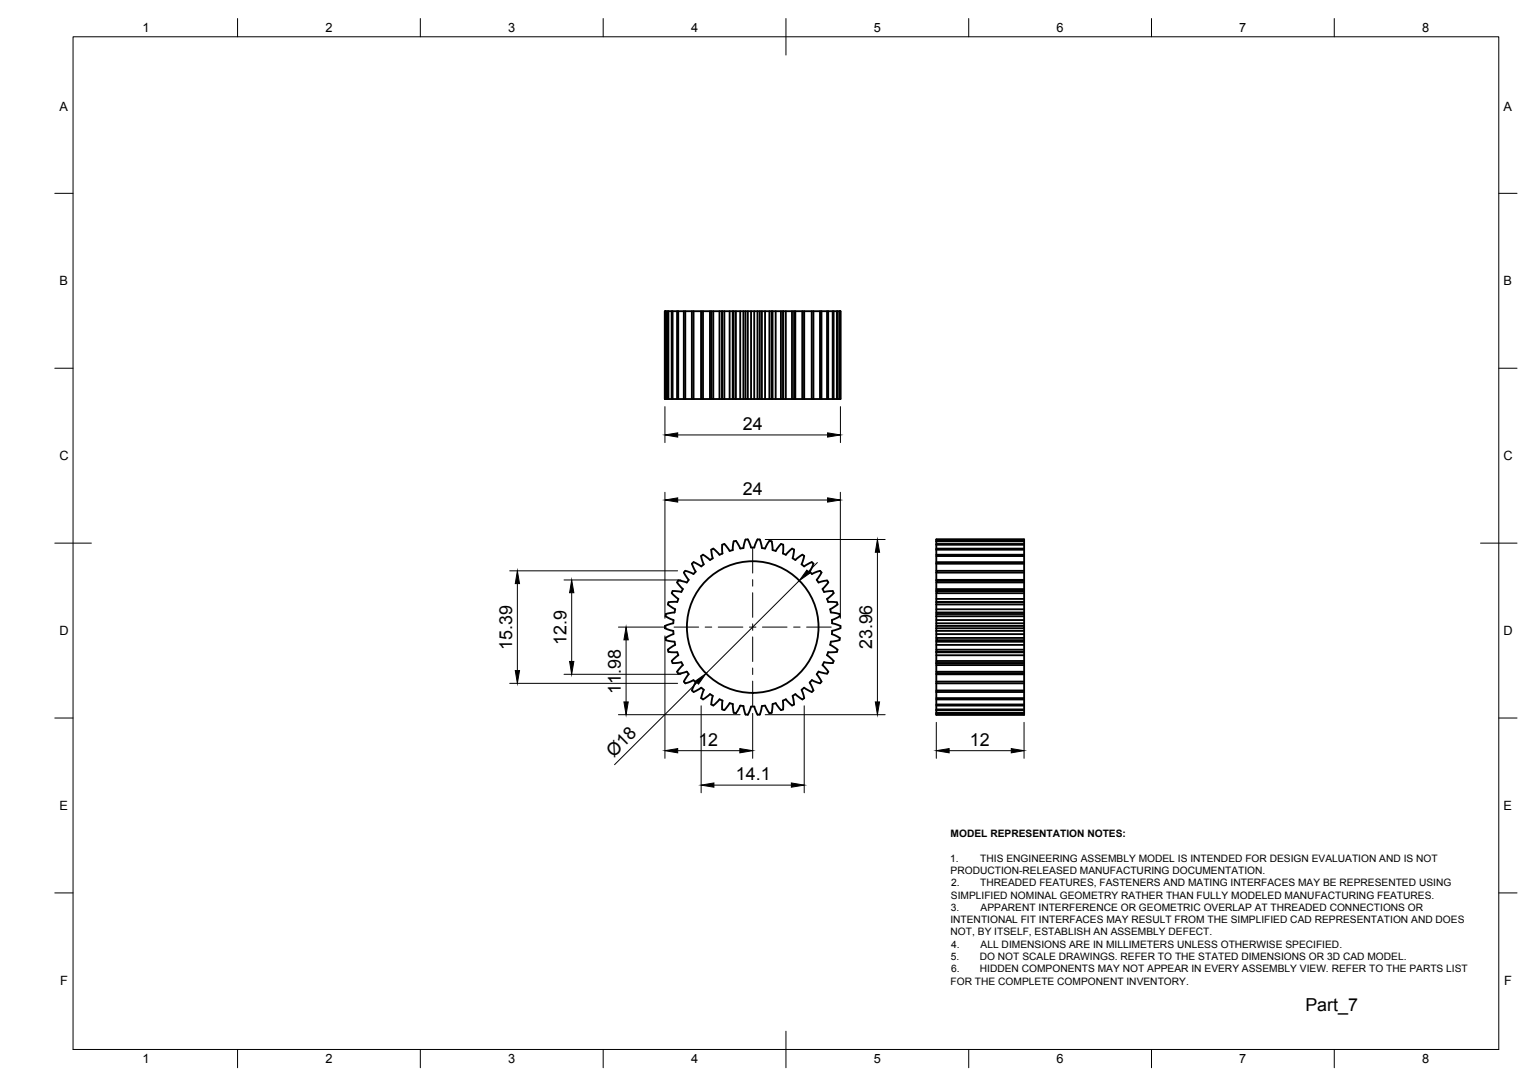
ISO-10303-21;
HEADER;
/* Generated by software containing ST-Developer
 * from STEP Tools, Inc. (www.steptools.com) 
 */

FILE_DESCRIPTION(
/* description */ ('STEP AP242 Edition 2'),
/* implementation_level */ '2;1');

FILE_NAME(
/* name */ 'Part_7.step',
/* time_stamp */ '2026-10-06T10:11:12-07:00',
/* author */ (''),
/* organization */ (''),
/* preprocessor_version */ 'ST-DEVELOPER v20.2',
/* originating_system */ 'Autodesk Translation Framework v15.15.0.0',
/* authorisation */ '');

FILE_SCHEMA (('AUTOMOTIVE_DESIGN { 1 0 10303 214 3 1 1 }'));
ENDSEC;

DATA;
#10=MECHANICAL_DESIGN_GEOMETRIC_PRESENTATION_REPRESENTATION('',(#1771),#54580);
#1743=SHAPE_REPRESENTATION_RELATIONSHIP('SRR','None',#54630,#1757);
#1757=ADVANCED_BREP_SHAPE_REPRESENTATION('',(#1801),#54566);
#1771=STYLED_ITEM('',(#54709),#1801);
#1801=MANIFOLD_SOLID_BREP('Body1',#17666);
#1815=LINE('',#24101,#2408);
#1816=LINE('',#24103,#2409);
#1817=LINE('',#24107,#2410);
#1818=LINE('',#24110,#2411);
#1819=LINE('',#24113,#2412);
#1820=LINE('',#24115,#2413);
#1821=LINE('',#24119,#2414);
#1822=LINE('',#24121,#2415);
#1823=LINE('',#24125,#2416);
#1824=LINE('',#24127,#2417);
#1825=LINE('',#24131,#2418);
#1826=LINE('',#24134,#2419);
#1827=LINE('',#24137,#2420);
#1828=LINE('',#24140,#2421);
#1829=LINE('',#24143,#2422);
#1830=LINE('',#24145,#2423);
#1831=LINE('',#24149,#2424);
#1832=LINE('',#24152,#2425);
#1833=LINE('',#24155,#2426);
#1834=LINE('',#24157,#2427);
#1835=LINE('',#24161,#2428);
#1836=LINE('',#24163,#2429);
#1837=LINE('',#24167,#2430);
#1838=LINE('',#24169,#2431);
#1839=LINE('',#24173,#2432);
#1840=LINE('',#24175,#2433);
#1841=LINE('',#24179,#2434);
#1842=LINE('',#24182,#2435);
#1843=LINE('',#24185,#2436);
#1844=LINE('',#24187,#2437);
#1845=LINE('',#24191,#2438);
#1846=LINE('',#24193,#2439);
#1847=LINE('',#24197,#2440);
#1848=LINE('',#24199,#2441);
#1849=LINE('',#24203,#2442);
#1850=LINE('',#24206,#2443);
#1851=LINE('',#24209,#2444);
#1852=LINE('',#24212,#2445);
#1853=LINE('',#24215,#2446);
#1854=LINE('',#24217,#2447);
#1855=LINE('',#24221,#2448);
#1856=LINE('',#24224,#2449);
#1857=LINE('',#24227,#2450);
#1858=LINE('',#24229,#2451);
#1859=LINE('',#24233,#2452);
#1860=LINE('',#24235,#2453);
#1861=LINE('',#24239,#2454);
#1862=LINE('',#24241,#2455);
#1863=LINE('',#24245,#2456);
#1864=LINE('',#24248,#2457);
#1865=LINE('',#24251,#2458);
#1866=LINE('',#24253,#2459);
#1867=LINE('',#24257,#2460);
#1868=LINE('',#24259,#2461);
#1869=LINE('',#24263,#2462);
#1870=LINE('',#24265,#2463);
#1871=LINE('',#24269,#2464);
#1872=LINE('',#24272,#2465);
#1873=LINE('',#24275,#2466);
#1874=LINE('',#24277,#2467);
#1875=LINE('',#24281,#2468);
#1876=LINE('',#24283,#2469);
#1877=LINE('',#24287,#2470);
#1878=LINE('',#24290,#2471);
#1879=LINE('',#24293,#2472);
#1880=LINE('',#24295,#2473);
#1881=LINE('',#24299,#2474);
#1882=LINE('',#24301,#2475);
#1883=LINE('',#24305,#2476);
#1884=LINE('',#24307,#2477);
#1885=LINE('',#24311,#2478);
#1886=LINE('',#24314,#2479);
#1887=LINE('',#24317,#2480);
#1888=LINE('',#24319,#2481);
#1889=LINE('',#24323,#2482);
#1890=LINE('',#24325,#2483);
#1891=LINE('',#24329,#2484);
#1892=LINE('',#24331,#2485);
#1893=LINE('',#24335,#2486);
#1894=LINE('',#24338,#2487);
#1895=LINE('',#24341,#2488);
#1896=LINE('',#24343,#2489);
#1897=LINE('',#24347,#2490);
#1898=LINE('',#24349,#2491);
#1899=LINE('',#24353,#2492);
#1900=LINE('',#24356,#2493);
#1901=LINE('',#24359,#2494);
#1902=LINE('',#24361,#2495);
#1903=LINE('',#24365,#2496);
#1904=LINE('',#24367,#2497);
#1905=LINE('',#24606,#2498);
#1906=LINE('',#24607,#2499);
#1907=LINE('',#24609,#2500);
#1908=LINE('',#24611,#2501);
#1909=LINE('',#24614,#2502);
#1910=LINE('',#24616,#2503);
#1911=LINE('',#24619,#2504);
#1912=LINE('',#24621,#2505);
#1913=LINE('',#24624,#2506);
#1914=LINE('',#24626,#2507);
#1915=LINE('',#24629,#2508);
#1916=LINE('',#24631,#2509);
#1917=LINE('',#24634,#2510);
#1918=LINE('',#24636,#2511);
#1919=LINE('',#24639,#2512);
#1920=LINE('',#24641,#2513);
#1921=LINE('',#24644,#2514);
#1922=LINE('',#24646,#2515);
#1923=LINE('',#24649,#2516);
#1924=LINE('',#24651,#2517);
#1925=LINE('',#24654,#2518);
#1926=LINE('',#24656,#2519);
#1927=LINE('',#24659,#2520);
#1928=LINE('',#24661,#2521);
#1929=LINE('',#24664,#2522);
#1930=LINE('',#24666,#2523);
#1931=LINE('',#24669,#2524);
#1932=LINE('',#24671,#2525);
#1933=LINE('',#24674,#2526);
#1934=LINE('',#24676,#2527);
#1935=LINE('',#24679,#2528);
#1936=LINE('',#24681,#2529);
#1937=LINE('',#24684,#2530);
#1938=LINE('',#24686,#2531);
#1939=LINE('',#24689,#2532);
#1940=LINE('',#24691,#2533);
#1941=LINE('',#24694,#2534);
#1942=LINE('',#24696,#2535);
#1943=LINE('',#24699,#2536);
#1944=LINE('',#24701,#2537);
#1945=LINE('',#24704,#2538);
#1946=LINE('',#24706,#2539);
#1947=LINE('',#24709,#2540);
#1948=LINE('',#24711,#2541);
#1949=LINE('',#24714,#2542);
#1950=LINE('',#24716,#2543);
#1951=LINE('',#24719,#2544);
#1952=LINE('',#24721,#2545);
#1953=LINE('',#24724,#2546);
#1954=LINE('',#24726,#2547);
#1955=LINE('',#24729,#2548);
#1956=LINE('',#24731,#2549);
#1957=LINE('',#24734,#2550);
#1958=LINE('',#24736,#2551);
#1959=LINE('',#24739,#2552);
#1960=LINE('',#24741,#2553);
#1961=LINE('',#24744,#2554);
#1962=LINE('',#24746,#2555);
#1963=LINE('',#24749,#2556);
#1964=LINE('',#24751,#2557);
#1965=LINE('',#24754,#2558);
#1966=LINE('',#24756,#2559);
#1967=LINE('',#24759,#2560);
#1968=LINE('',#24761,#2561);
#1969=LINE('',#24764,#2562);
#1970=LINE('',#24766,#2563);
#1971=LINE('',#24769,#2564);
#1972=LINE('',#24771,#2565);
#1973=LINE('',#24774,#2566);
#1974=LINE('',#24776,#2567);
#1975=LINE('',#24779,#2568);
#1976=LINE('',#24781,#2569);
#1977=LINE('',#24784,#2570);
#1978=LINE('',#24786,#2571);
#1979=LINE('',#24789,#2572);
#1980=LINE('',#24791,#2573);
#1981=LINE('',#24794,#2574);
#1982=LINE('',#24796,#2575);
#1983=LINE('',#24799,#2576);
#1984=LINE('',#24801,#2577);
#1985=LINE('',#24804,#2578);
#1986=LINE('',#24806,#2579);
#1987=LINE('',#24809,#2580);
#1988=LINE('',#24811,#2581);
#1989=LINE('',#24814,#2582);
#1990=LINE('',#24816,#2583);
#1991=LINE('',#24819,#2584);
#1992=LINE('',#24821,#2585);
#1993=LINE('',#24824,#2586);
#1994=LINE('',#24826,#2587);
#1995=LINE('',#24829,#2588);
#1996=LINE('',#24831,#2589);
#1997=LINE('',#24834,#2590);
#1998=LINE('',#24836,#2591);
#1999=LINE('',#24839,#2592);
#2408=VECTOR('',#19979,1.);
#2409=VECTOR('',#19980,1.);
#2410=VECTOR('',#19985,1.);
#2411=VECTOR('',#19988,1.);
#2412=VECTOR('',#19991,1.);
#2413=VECTOR('',#19992,1.);
#2414=VECTOR('',#19997,1.);
#2415=VECTOR('',#19998,1.);
#2416=VECTOR('',#20003,1.);
#2417=VECTOR('',#20004,1.);
#2418=VECTOR('',#20009,1.);
#2419=VECTOR('',#20012,1.);
#2420=VECTOR('',#20015,1.);
#2421=VECTOR('',#20018,1.);
#2422=VECTOR('',#20021,1.);
#2423=VECTOR('',#20022,1.);
#2424=VECTOR('',#20027,1.);
#2425=VECTOR('',#20030,1.);
#2426=VECTOR('',#20033,1.);
#2427=VECTOR('',#20034,1.);
#2428=VECTOR('',#20039,1.);
#2429=VECTOR('',#20040,1.);
#2430=VECTOR('',#20045,1.);
#2431=VECTOR('',#20046,1.);
#2432=VECTOR('',#20051,1.);
#2433=VECTOR('',#20052,1.);
#2434=VECTOR('',#20057,1.);
#2435=VECTOR('',#20060,1.);
#2436=VECTOR('',#20063,1.);
#2437=VECTOR('',#20064,1.);
#2438=VECTOR('',#20069,1.);
#2439=VECTOR('',#20070,1.);
#2440=VECTOR('',#20075,1.);
#2441=VECTOR('',#20076,1.);
#2442=VECTOR('',#20081,1.);
#2443=VECTOR('',#20084,1.);
#2444=VECTOR('',#20087,1.);
#2445=VECTOR('',#20090,1.);
#2446=VECTOR('',#20093,1.);
#2447=VECTOR('',#20094,1.);
#2448=VECTOR('',#20099,1.);
#2449=VECTOR('',#20102,1.);
#2450=VECTOR('',#20105,1.);
#2451=VECTOR('',#20106,1.);
#2452=VECTOR('',#20111,1.);
#2453=VECTOR('',#20112,1.);
#2454=VECTOR('',#20117,1.);
#2455=VECTOR('',#20118,1.);
#2456=VECTOR('',#20123,1.);
#2457=VECTOR('',#20126,1.);
#2458=VECTOR('',#20129,1.);
#2459=VECTOR('',#20130,1.);
#2460=VECTOR('',#20135,1.);
#2461=VECTOR('',#20136,1.);
#2462=VECTOR('',#20141,1.);
#2463=VECTOR('',#20142,1.);
#2464=VECTOR('',#20147,1.);
#2465=VECTOR('',#20150,1.);
#2466=VECTOR('',#20153,1.);
#2467=VECTOR('',#20154,1.);
#2468=VECTOR('',#20159,1.);
#2469=VECTOR('',#20160,1.);
#2470=VECTOR('',#20165,1.);
#2471=VECTOR('',#20168,1.);
#2472=VECTOR('',#20171,1.);
#2473=VECTOR('',#20172,1.);
#2474=VECTOR('',#20177,1.);
#2475=VECTOR('',#20178,1.);
#2476=VECTOR('',#20183,1.);
#2477=VECTOR('',#20184,1.);
#2478=VECTOR('',#20189,1.);
#2479=VECTOR('',#20192,1.);
#2480=VECTOR('',#20195,1.);
#2481=VECTOR('',#20196,1.);
#2482=VECTOR('',#20201,1.);
#2483=VECTOR('',#20202,1.);
#2484=VECTOR('',#20207,1.);
#2485=VECTOR('',#20208,1.);
#2486=VECTOR('',#20213,1.);
#2487=VECTOR('',#20216,1.);
#2488=VECTOR('',#20219,1.);
#2489=VECTOR('',#20220,1.);
#2490=VECTOR('',#20225,1.);
#2491=VECTOR('',#20226,1.);
#2492=VECTOR('',#20231,1.);
#2493=VECTOR('',#20234,1.);
#2494=VECTOR('',#20237,1.);
#2495=VECTOR('',#20238,1.);
#2496=VECTOR('',#20243,1.);
#2497=VECTOR('',#20244,1.);
#2498=VECTOR('',#20531,1.);
#2499=VECTOR('',#20532,1.);
#2500=VECTOR('',#20535,1.);
#2501=VECTOR('',#20538,1.);
#2502=VECTOR('',#20543,1.);
#2503=VECTOR('',#20546,1.);
#2504=VECTOR('',#20551,1.);
#2505=VECTOR('',#20554,1.);
#2506=VECTOR('',#20559,1.);
#2507=VECTOR('',#20562,1.);
#2508=VECTOR('',#20567,1.);
#2509=VECTOR('',#20570,1.);
#2510=VECTOR('',#20575,1.);
#2511=VECTOR('',#20578,1.);
#2512=VECTOR('',#20583,1.);
#2513=VECTOR('',#20586,1.);
#2514=VECTOR('',#20591,1.);
#2515=VECTOR('',#20594,1.);
#2516=VECTOR('',#20599,1.);
#2517=VECTOR('',#20602,1.);
#2518=VECTOR('',#20607,1.);
#2519=VECTOR('',#20610,1.);
#2520=VECTOR('',#20615,1.);
#2521=VECTOR('',#20618,1.);
#2522=VECTOR('',#20623,1.);
#2523=VECTOR('',#20626,1.);
#2524=VECTOR('',#20631,1.);
#2525=VECTOR('',#20634,1.);
#2526=VECTOR('',#20639,1.);
#2527=VECTOR('',#20642,1.);
#2528=VECTOR('',#20647,1.);
#2529=VECTOR('',#20650,1.);
#2530=VECTOR('',#20655,1.);
#2531=VECTOR('',#20658,1.);
#2532=VECTOR('',#20663,1.);
#2533=VECTOR('',#20666,1.);
#2534=VECTOR('',#20671,1.);
#2535=VECTOR('',#20674,1.);
#2536=VECTOR('',#20679,1.);
#2537=VECTOR('',#20682,1.);
#2538=VECTOR('',#20687,1.);
#2539=VECTOR('',#20690,1.);
#2540=VECTOR('',#20695,1.);
#2541=VECTOR('',#20698,1.);
#2542=VECTOR('',#20703,1.);
#2543=VECTOR('',#20706,1.);
#2544=VECTOR('',#20711,1.);
#2545=VECTOR('',#20714,1.);
#2546=VECTOR('',#20719,1.);
#2547=VECTOR('',#20722,1.);
#2548=VECTOR('',#20727,1.);
#2549=VECTOR('',#20730,1.);
#2550=VECTOR('',#20735,1.);
#2551=VECTOR('',#20738,1.);
#2552=VECTOR('',#20743,1.);
#2553=VECTOR('',#20746,1.);
#2554=VECTOR('',#20751,1.);
#2555=VECTOR('',#20754,1.);
#2556=VECTOR('',#20759,1.);
#2557=VECTOR('',#20762,1.);
#2558=VECTOR('',#20767,1.);
#2559=VECTOR('',#20770,1.);
#2560=VECTOR('',#20775,1.);
#2561=VECTOR('',#20778,1.);
#2562=VECTOR('',#20783,1.);
#2563=VECTOR('',#20786,1.);
#2564=VECTOR('',#20791,1.);
#2565=VECTOR('',#20794,1.);
#2566=VECTOR('',#20799,1.);
#2567=VECTOR('',#20802,1.);
#2568=VECTOR('',#20807,1.);
#2569=VECTOR('',#20810,1.);
#2570=VECTOR('',#20815,1.);
#2571=VECTOR('',#20818,1.);
#2572=VECTOR('',#20823,1.);
#2573=VECTOR('',#20826,1.);
#2574=VECTOR('',#20831,1.);
#2575=VECTOR('',#20834,1.);
#2576=VECTOR('',#20839,1.);
#2577=VECTOR('',#20842,1.);
#2578=VECTOR('',#20847,1.);
#2579=VECTOR('',#20850,1.);
#2580=VECTOR('',#20855,1.);
#2581=VECTOR('',#20858,1.);
#2582=VECTOR('',#20863,1.);
#2583=VECTOR('',#20866,1.);
#2584=VECTOR('',#20871,1.);
#2585=VECTOR('',#20874,1.);
#2586=VECTOR('',#20879,1.);
#2587=VECTOR('',#20882,1.);
#2588=VECTOR('',#20887,1.);
#2589=VECTOR('',#20890,1.);
#2590=VECTOR('',#20895,1.);
#2591=VECTOR('',#20898,1.);
#2592=VECTOR('',#20903,0.009);
#3001=CYLINDRICAL_SURFACE('',#18023,0.012);
#3002=CYLINDRICAL_SURFACE('',#18025,0.012);
#3003=CYLINDRICAL_SURFACE('',#18027,0.012);
#3004=CYLINDRICAL_SURFACE('',#18029,0.012);
#3005=CYLINDRICAL_SURFACE('',#18031,0.012);
#3006=CYLINDRICAL_SURFACE('',#18033,0.012);
#3007=CYLINDRICAL_SURFACE('',#18035,0.012);
#3008=CYLINDRICAL_SURFACE('',#18037,0.012);
#3009=CYLINDRICAL_SURFACE('',#18039,0.012);
#3010=CYLINDRICAL_SURFACE('',#18041,0.012);
#3011=CYLINDRICAL_SURFACE('',#18043,0.012);
#3012=CYLINDRICAL_SURFACE('',#18045,0.012);
#3013=CYLINDRICAL_SURFACE('',#18047,0.012);
#3014=CYLINDRICAL_SURFACE('',#18049,0.012);
#3015=CYLINDRICAL_SURFACE('',#18051,0.012);
#3016=CYLINDRICAL_SURFACE('',#18053,0.012);
#3017=CYLINDRICAL_SURFACE('',#18055,0.012);
#3018=CYLINDRICAL_SURFACE('',#18057,0.012);
#3019=CYLINDRICAL_SURFACE('',#18059,0.012);
#3020=CYLINDRICAL_SURFACE('',#18061,0.012);
#3021=CYLINDRICAL_SURFACE('',#18063,0.012);
#3022=CYLINDRICAL_SURFACE('',#18065,0.012);
#3023=CYLINDRICAL_SURFACE('',#18067,0.012);
#3024=CYLINDRICAL_SURFACE('',#18069,0.012);
#3025=CYLINDRICAL_SURFACE('',#18071,0.012);
#3026=CYLINDRICAL_SURFACE('',#18073,0.012);
#3027=CYLINDRICAL_SURFACE('',#18075,0.012);
#3028=CYLINDRICAL_SURFACE('',#18077,0.012);
#3029=CYLINDRICAL_SURFACE('',#18079,0.012);
#3030=CYLINDRICAL_SURFACE('',#18081,0.012);
#3031=CYLINDRICAL_SURFACE('',#18083,0.012);
#3032=CYLINDRICAL_SURFACE('',#18085,0.012);
#3033=CYLINDRICAL_SURFACE('',#18087,0.012);
#3034=CYLINDRICAL_SURFACE('',#18089,0.012);
#3035=CYLINDRICAL_SURFACE('',#18091,0.012);
#3036=CYLINDRICAL_SURFACE('',#18093,0.012);
#3037=CYLINDRICAL_SURFACE('',#18095,0.012);
#3038=CYLINDRICAL_SURFACE('',#18097,0.012);
#3039=CYLINDRICAL_SURFACE('',#18099,0.012);
#3040=CYLINDRICAL_SURFACE('',#18101,0.012);
#3041=CYLINDRICAL_SURFACE('',#18103,0.012);
#3042=CYLINDRICAL_SURFACE('',#18105,0.012);
#3043=CYLINDRICAL_SURFACE('',#18107,0.012);
#3044=CYLINDRICAL_SURFACE('',#18109,0.012);
#3045=CYLINDRICAL_SURFACE('',#18111,0.012);
#3046=CYLINDRICAL_SURFACE('',#18254,0.012);
#3047=CYLINDRICAL_SURFACE('',#18255,0.0046);
#3048=CYLINDRICAL_SURFACE('',#18256,0.0046);
#3049=CYLINDRICAL_SURFACE('',#18257,0.010874);
#3050=CYLINDRICAL_SURFACE('',#18258,0.0046);
#3051=CYLINDRICAL_SURFACE('',#18259,0.0046);
#3052=CYLINDRICAL_SURFACE('',#18260,0.010874);
#3053=CYLINDRICAL_SURFACE('',#18261,0.0046);
#3054=CYLINDRICAL_SURFACE('',#18262,0.0046);
#3055=CYLINDRICAL_SURFACE('',#18263,0.010874);
#3056=CYLINDRICAL_SURFACE('',#18264,0.0046);
#3057=CYLINDRICAL_SURFACE('',#18265,0.0046);
#3058=CYLINDRICAL_SURFACE('',#18266,0.010874);
#3059=CYLINDRICAL_SURFACE('',#18267,0.0046);
#3060=CYLINDRICAL_SURFACE('',#18268,0.0046);
#3061=CYLINDRICAL_SURFACE('',#18269,0.010874);
#3062=CYLINDRICAL_SURFACE('',#18270,0.0046);
#3063=CYLINDRICAL_SURFACE('',#18271,0.0046);
#3064=CYLINDRICAL_SURFACE('',#18272,0.010874);
#3065=CYLINDRICAL_SURFACE('',#18273,0.0046);
#3066=CYLINDRICAL_SURFACE('',#18274,0.0046);
#3067=CYLINDRICAL_SURFACE('',#18275,0.010874);
#3068=CYLINDRICAL_SURFACE('',#18276,0.0046);
#3069=CYLINDRICAL_SURFACE('',#18277,0.0046);
#3070=CYLINDRICAL_SURFACE('',#18278,0.010874);
#3071=CYLINDRICAL_SURFACE('',#18279,0.0046);
#3072=CYLINDRICAL_SURFACE('',#18280,0.0046);
#3073=CYLINDRICAL_SURFACE('',#18281,0.010874);
#3074=CYLINDRICAL_SURFACE('',#18282,0.0046);
#3075=CYLINDRICAL_SURFACE('',#18283,0.0046);
#3076=CYLINDRICAL_SURFACE('',#18284,0.010874);
#3077=CYLINDRICAL_SURFACE('',#18285,0.0046);
#3078=CYLINDRICAL_SURFACE('',#18286,0.0046);
#3079=CYLINDRICAL_SURFACE('',#18287,0.010874);
#3080=CYLINDRICAL_SURFACE('',#18288,0.0046);
#3081=CYLINDRICAL_SURFACE('',#18289,0.0046);
#3082=CYLINDRICAL_SURFACE('',#18290,0.010874);
#3083=CYLINDRICAL_SURFACE('',#18291,0.0046);
#3084=CYLINDRICAL_SURFACE('',#18292,0.0046);
#3085=CYLINDRICAL_SURFACE('',#18293,0.010874);
#3086=CYLINDRICAL_SURFACE('',#18294,0.0046);
#3087=CYLINDRICAL_SURFACE('',#18295,0.0046);
#3088=CYLINDRICAL_SURFACE('',#18296,0.010874);
#3089=CYLINDRICAL_SURFACE('',#18297,0.0046);
#3090=CYLINDRICAL_SURFACE('',#18298,0.0046);
#3091=CYLINDRICAL_SURFACE('',#18299,0.010874);
#3092=CYLINDRICAL_SURFACE('',#18300,0.0046);
#3093=CYLINDRICAL_SURFACE('',#18301,0.0046);
#3094=CYLINDRICAL_SURFACE('',#18302,0.010874);
#3095=CYLINDRICAL_SURFACE('',#18303,0.0046);
#3096=CYLINDRICAL_SURFACE('',#18304,0.0046);
#3097=CYLINDRICAL_SURFACE('',#18305,0.010874);
#3098=CYLINDRICAL_SURFACE('',#18306,0.0046);
#3099=CYLINDRICAL_SURFACE('',#18307,0.0046);
#3100=CYLINDRICAL_SURFACE('',#18308,0.010874);
#3101=CYLINDRICAL_SURFACE('',#18309,0.0046);
#3102=CYLINDRICAL_SURFACE('',#18310,0.0046);
#3103=CYLINDRICAL_SURFACE('',#18311,0.010874);
#3104=CYLINDRICAL_SURFACE('',#18312,0.0046);
#3105=CYLINDRICAL_SURFACE('',#18313,0.0046);
#3106=CYLINDRICAL_SURFACE('',#18314,0.010874);
#3107=CYLINDRICAL_SURFACE('',#18315,0.0046);
#3108=CYLINDRICAL_SURFACE('',#18316,0.0046);
#3109=CYLINDRICAL_SURFACE('',#18317,0.010874);
#3110=CYLINDRICAL_SURFACE('',#18318,0.0046);
#3111=CYLINDRICAL_SURFACE('',#18319,0.0046);
#3112=CYLINDRICAL_SURFACE('',#18320,0.010874);
#3113=CYLINDRICAL_SURFACE('',#18321,0.0046);
#3114=CYLINDRICAL_SURFACE('',#18322,0.0046);
#3115=CYLINDRICAL_SURFACE('',#18323,0.010874);
#3116=CYLINDRICAL_SURFACE('',#18324,0.0046);
#3117=CYLINDRICAL_SURFACE('',#18325,0.0046);
#3118=CYLINDRICAL_SURFACE('',#18326,0.010874);
#3119=CYLINDRICAL_SURFACE('',#18327,0.0046);
#3120=CYLINDRICAL_SURFACE('',#18328,0.0046);
#3121=CYLINDRICAL_SURFACE('',#18329,0.010874);
#3122=CYLINDRICAL_SURFACE('',#18330,0.0046);
#3123=CYLINDRICAL_SURFACE('',#18331,0.0046);
#3124=CYLINDRICAL_SURFACE('',#18332,0.010874);
#3125=CYLINDRICAL_SURFACE('',#18333,0.0046);
#3126=CYLINDRICAL_SURFACE('',#18334,0.0046);
#3127=CYLINDRICAL_SURFACE('',#18335,0.010874);
#3128=CYLINDRICAL_SURFACE('',#18336,0.0046);
#3129=CYLINDRICAL_SURFACE('',#18337,0.0046);
#3130=CYLINDRICAL_SURFACE('',#18338,0.010874);
#3131=CYLINDRICAL_SURFACE('',#18339,0.0046);
#3132=CYLINDRICAL_SURFACE('',#18340,0.0046);
#3133=CYLINDRICAL_SURFACE('',#18341,0.010874);
#3134=CYLINDRICAL_SURFACE('',#18342,0.0046);
#3135=CYLINDRICAL_SURFACE('',#18343,0.0046);
#3136=CYLINDRICAL_SURFACE('',#18344,0.010874);
#3137=CYLINDRICAL_SURFACE('',#18345,0.0046);
#3138=CYLINDRICAL_SURFACE('',#18346,0.0046);
#3139=CYLINDRICAL_SURFACE('',#18347,0.010874);
#3140=CYLINDRICAL_SURFACE('',#18348,0.0046);
#3141=CYLINDRICAL_SURFACE('',#18349,0.0046);
#3142=CYLINDRICAL_SURFACE('',#18350,0.010874);
#3143=CYLINDRICAL_SURFACE('',#18351,0.0046);
#3144=CYLINDRICAL_SURFACE('',#18352,0.0046);
#3145=CYLINDRICAL_SURFACE('',#18353,0.010874);
#3146=CYLINDRICAL_SURFACE('',#18354,0.0046);
#3147=CYLINDRICAL_SURFACE('',#18355,0.0046);
#3148=CYLINDRICAL_SURFACE('',#18356,0.010874);
#3149=CYLINDRICAL_SURFACE('',#18357,0.0046);
#3150=CYLINDRICAL_SURFACE('',#18358,0.0046);
#3151=CYLINDRICAL_SURFACE('',#18359,0.010874);
#3152=CYLINDRICAL_SURFACE('',#18360,0.0046);
#3153=CYLINDRICAL_SURFACE('',#18361,0.0046);
#3154=CYLINDRICAL_SURFACE('',#18362,0.010874);
#3155=CYLINDRICAL_SURFACE('',#18363,0.0046);
#3156=CYLINDRICAL_SURFACE('',#18364,0.0046);
#3157=CYLINDRICAL_SURFACE('',#18365,0.010874);
#3158=CYLINDRICAL_SURFACE('',#18366,0.0046);
#3159=CYLINDRICAL_SURFACE('',#18367,0.0046);
#3160=CYLINDRICAL_SURFACE('',#18368,0.010874);
#3161=CYLINDRICAL_SURFACE('',#18369,0.0046);
#3162=CYLINDRICAL_SURFACE('',#18370,0.0046);
#3163=CYLINDRICAL_SURFACE('',#18371,0.010874);
#3164=CYLINDRICAL_SURFACE('',#18372,0.0046);
#3165=CYLINDRICAL_SURFACE('',#18373,0.0046);
#3166=CYLINDRICAL_SURFACE('',#18374,0.010874);
#3167=CYLINDRICAL_SURFACE('',#18375,0.0046);
#3168=CYLINDRICAL_SURFACE('',#18376,0.0046);
#3169=CYLINDRICAL_SURFACE('',#18377,0.010874);
#3170=CYLINDRICAL_SURFACE('',#18378,0.0046);
#3171=CYLINDRICAL_SURFACE('',#18379,0.0046);
#3172=CYLINDRICAL_SURFACE('',#18380,0.010874);
#3173=CYLINDRICAL_SURFACE('',#18381,0.0046);
#3174=CYLINDRICAL_SURFACE('',#18382,0.0046);
#3175=CYLINDRICAL_SURFACE('',#18383,0.010874);
#3176=CYLINDRICAL_SURFACE('',#18384,0.0046);
#3177=CYLINDRICAL_SURFACE('',#18385,0.0046);
#3178=CYLINDRICAL_SURFACE('',#18386,0.010874);
#3179=CYLINDRICAL_SURFACE('',#18387,0.0046);
#3180=CYLINDRICAL_SURFACE('',#18388,0.0046);
#3181=CYLINDRICAL_SURFACE('',#18389,0.010874);
#3182=CYLINDRICAL_SURFACE('',#18390,0.0046);
#3183=CYLINDRICAL_SURFACE('',#18391,0.0046);
#3184=CYLINDRICAL_SURFACE('',#18392,0.010874);
#3185=CYLINDRICAL_SURFACE('',#18393,0.009);
#3477=FACE_BOUND('',#4551,.T.);
#3478=FACE_BOUND('',#4598,.T.);
#3544=FACE_OUTER_BOUND('',#4550,.T.);
#3545=FACE_OUTER_BOUND('',#4552,.T.);
#3546=FACE_OUTER_BOUND('',#4553,.T.);
#3547=FACE_OUTER_BOUND('',#4554,.T.);
#3548=FACE_OUTER_BOUND('',#4555,.T.);
#3549=FACE_OUTER_BOUND('',#4556,.T.);
#3550=FACE_OUTER_BOUND('',#4557,.T.);
#3551=FACE_OUTER_BOUND('',#4558,.T.);
#3552=FACE_OUTER_BOUND('',#4559,.T.);
#3553=FACE_OUTER_BOUND('',#4560,.T.);
#3554=FACE_OUTER_BOUND('',#4561,.T.);
#3555=FACE_OUTER_BOUND('',#4562,.T.);
#3556=FACE_OUTER_BOUND('',#4563,.T.);
#3557=FACE_OUTER_BOUND('',#4564,.T.);
#3558=FACE_OUTER_BOUND('',#4565,.T.);
#3559=FACE_OUTER_BOUND('',#4566,.T.);
#3560=FACE_OUTER_BOUND('',#4567,.T.);
#3561=FACE_OUTER_BOUND('',#4568,.T.);
#3562=FACE_OUTER_BOUND('',#4569,.T.);
#3563=FACE_OUTER_BOUND('',#4570,.T.);
#3564=FACE_OUTER_BOUND('',#4571,.T.);
#3565=FACE_OUTER_BOUND('',#4572,.T.);
#3566=FACE_OUTER_BOUND('',#4573,.T.);
#3567=FACE_OUTER_BOUND('',#4574,.T.);
#3568=FACE_OUTER_BOUND('',#4575,.T.);
#3569=FACE_OUTER_BOUND('',#4576,.T.);
#3570=FACE_OUTER_BOUND('',#4577,.T.);
#3571=FACE_OUTER_BOUND('',#4578,.T.);
#3572=FACE_OUTER_BOUND('',#4579,.T.);
#3573=FACE_OUTER_BOUND('',#4580,.T.);
#3574=FACE_OUTER_BOUND('',#4581,.T.);
#3575=FACE_OUTER_BOUND('',#4582,.T.);
#3576=FACE_OUTER_BOUND('',#4583,.T.);
#3577=FACE_OUTER_BOUND('',#4584,.T.);
#3578=FACE_OUTER_BOUND('',#4585,.T.);
#3579=FACE_OUTER_BOUND('',#4586,.T.);
#3580=FACE_OUTER_BOUND('',#4587,.T.);
#3581=FACE_OUTER_BOUND('',#4588,.T.);
#3582=FACE_OUTER_BOUND('',#4589,.T.);
#3583=FACE_OUTER_BOUND('',#4590,.T.);
#3584=FACE_OUTER_BOUND('',#4591,.T.);
#3585=FACE_OUTER_BOUND('',#4592,.T.);
#3586=FACE_OUTER_BOUND('',#4593,.T.);
#3587=FACE_OUTER_BOUND('',#4594,.T.);
#3588=FACE_OUTER_BOUND('',#4595,.T.);
#3589=FACE_OUTER_BOUND('',#4596,.T.);
#3590=FACE_OUTER_BOUND('',#4597,.T.);
#3591=FACE_OUTER_BOUND('',#4599,.T.);
#3592=FACE_OUTER_BOUND('',#4600,.T.);
#3593=FACE_OUTER_BOUND('',#4601,.T.);
#3594=FACE_OUTER_BOUND('',#4602,.T.);
#3595=FACE_OUTER_BOUND('',#4603,.T.);
#3596=FACE_OUTER_BOUND('',#4604,.T.);
#3597=FACE_OUTER_BOUND('',#4605,.T.);
#3598=FACE_OUTER_BOUND('',#4606,.T.);
#3599=FACE_OUTER_BOUND('',#4607,.T.);
#3600=FACE_OUTER_BOUND('',#4608,.T.);
#3601=FACE_OUTER_BOUND('',#4609,.T.);
#3602=FACE_OUTER_BOUND('',#4610,.T.);
#3603=FACE_OUTER_BOUND('',#4611,.T.);
#3604=FACE_OUTER_BOUND('',#4612,.T.);
#3605=FACE_OUTER_BOUND('',#4613,.T.);
#3606=FACE_OUTER_BOUND('',#4614,.T.);
#3607=FACE_OUTER_BOUND('',#4615,.T.);
#3608=FACE_OUTER_BOUND('',#4616,.T.);
#3609=FACE_OUTER_BOUND('',#4617,.T.);
#3610=FACE_OUTER_BOUND('',#4618,.T.);
#3611=FACE_OUTER_BOUND('',#4619,.T.);
#3612=FACE_OUTER_BOUND('',#4620,.T.);
#3613=FACE_OUTER_BOUND('',#4621,.T.);
#3614=FACE_OUTER_BOUND('',#4622,.T.);
#3615=FACE_OUTER_BOUND('',#4623,.T.);
#3616=FACE_OUTER_BOUND('',#4624,.T.);
#3617=FACE_OUTER_BOUND('',#4625,.T.);
#3618=FACE_OUTER_BOUND('',#4626,.T.);
#3619=FACE_OUTER_BOUND('',#4627,.T.);
#3620=FACE_OUTER_BOUND('',#4628,.T.);
#3621=FACE_OUTER_BOUND('',#4629,.T.);
#3622=FACE_OUTER_BOUND('',#4630,.T.);
#3623=FACE_OUTER_BOUND('',#4631,.T.);
#3624=FACE_OUTER_BOUND('',#4632,.T.);
#3625=FACE_OUTER_BOUND('',#4633,.T.);
#3626=FACE_OUTER_BOUND('',#4634,.T.);
#3627=FACE_OUTER_BOUND('',#4635,.T.);
#3628=FACE_OUTER_BOUND('',#4636,.T.);
#3629=FACE_OUTER_BOUND('',#4637,.T.);
#3630=FACE_OUTER_BOUND('',#4638,.T.);
#3631=FACE_OUTER_BOUND('',#4639,.T.);
#3632=FACE_OUTER_BOUND('',#4640,.T.);
#3633=FACE_OUTER_BOUND('',#4641,.T.);
#3634=FACE_OUTER_BOUND('',#4642,.T.);
#3635=FACE_OUTER_BOUND('',#4643,.T.);
#3636=FACE_OUTER_BOUND('',#4644,.T.);
#3637=FACE_OUTER_BOUND('',#4645,.T.);
#3638=FACE_OUTER_BOUND('',#4646,.T.);
#3639=FACE_OUTER_BOUND('',#4647,.T.);
#3640=FACE_OUTER_BOUND('',#4648,.T.);
#3641=FACE_OUTER_BOUND('',#4649,.T.);
#3642=FACE_OUTER_BOUND('',#4650,.T.);
#3643=FACE_OUTER_BOUND('',#4651,.T.);
#3644=FACE_OUTER_BOUND('',#4652,.T.);
#3645=FACE_OUTER_BOUND('',#4653,.T.);
#3646=FACE_OUTER_BOUND('',#4654,.T.);
#3647=FACE_OUTER_BOUND('',#4655,.T.);
#3648=FACE_OUTER_BOUND('',#4656,.T.);
#3649=FACE_OUTER_BOUND('',#4657,.T.);
#3650=FACE_OUTER_BOUND('',#4658,.T.);
#3651=FACE_OUTER_BOUND('',#4659,.T.);
#3652=FACE_OUTER_BOUND('',#4660,.T.);
#3653=FACE_OUTER_BOUND('',#4661,.T.);
#3654=FACE_OUTER_BOUND('',#4662,.T.);
#3655=FACE_OUTER_BOUND('',#4663,.T.);
#3656=FACE_OUTER_BOUND('',#4664,.T.);
#3657=FACE_OUTER_BOUND('',#4665,.T.);
#3658=FACE_OUTER_BOUND('',#4666,.T.);
#3659=FACE_OUTER_BOUND('',#4667,.T.);
#3660=FACE_OUTER_BOUND('',#4668,.T.);
#3661=FACE_OUTER_BOUND('',#4669,.T.);
#3662=FACE_OUTER_BOUND('',#4670,.T.);
#3663=FACE_OUTER_BOUND('',#4671,.T.);
#3664=FACE_OUTER_BOUND('',#4672,.T.);
#3665=FACE_OUTER_BOUND('',#4673,.T.);
#3666=FACE_OUTER_BOUND('',#4674,.T.);
#3667=FACE_OUTER_BOUND('',#4675,.T.);
#3668=FACE_OUTER_BOUND('',#4676,.T.);
#3669=FACE_OUTER_BOUND('',#4677,.T.);
#3670=FACE_OUTER_BOUND('',#4678,.T.);
#3671=FACE_OUTER_BOUND('',#4679,.T.);
#3672=FACE_OUTER_BOUND('',#4680,.T.);
#3673=FACE_OUTER_BOUND('',#4681,.T.);
#3674=FACE_OUTER_BOUND('',#4682,.T.);
#3675=FACE_OUTER_BOUND('',#4683,.T.);
#3676=FACE_OUTER_BOUND('',#4684,.T.);
#3677=FACE_OUTER_BOUND('',#4685,.T.);
#3678=FACE_OUTER_BOUND('',#4686,.T.);
#3679=FACE_OUTER_BOUND('',#4687,.T.);
#3680=FACE_OUTER_BOUND('',#4688,.T.);
#3681=FACE_OUTER_BOUND('',#4689,.T.);
#3682=FACE_OUTER_BOUND('',#4690,.T.);
#3683=FACE_OUTER_BOUND('',#4691,.T.);
#3684=FACE_OUTER_BOUND('',#4692,.T.);
#3685=FACE_OUTER_BOUND('',#4693,.T.);
#3686=FACE_OUTER_BOUND('',#4694,.T.);
#3687=FACE_OUTER_BOUND('',#4695,.T.);
#3688=FACE_OUTER_BOUND('',#4696,.T.);
#3689=FACE_OUTER_BOUND('',#4697,.T.);
#3690=FACE_OUTER_BOUND('',#4698,.T.);
#3691=FACE_OUTER_BOUND('',#4699,.T.);
#3692=FACE_OUTER_BOUND('',#4700,.T.);
#3693=FACE_OUTER_BOUND('',#4701,.T.);
#3694=FACE_OUTER_BOUND('',#4702,.T.);
#3695=FACE_OUTER_BOUND('',#4703,.T.);
#3696=FACE_OUTER_BOUND('',#4704,.T.);
#3697=FACE_OUTER_BOUND('',#4705,.T.);
#3698=FACE_OUTER_BOUND('',#4706,.T.);
#3699=FACE_OUTER_BOUND('',#4707,.T.);
#3700=FACE_OUTER_BOUND('',#4708,.T.);
#3701=FACE_OUTER_BOUND('',#4709,.T.);
#3702=FACE_OUTER_BOUND('',#4710,.T.);
#3703=FACE_OUTER_BOUND('',#4711,.T.);
#3704=FACE_OUTER_BOUND('',#4712,.T.);
#3705=FACE_OUTER_BOUND('',#4713,.T.);
#3706=FACE_OUTER_BOUND('',#4714,.T.);
#3707=FACE_OUTER_BOUND('',#4715,.T.);
#3708=FACE_OUTER_BOUND('',#4716,.T.);
#3709=FACE_OUTER_BOUND('',#4717,.T.);
#3710=FACE_OUTER_BOUND('',#4718,.T.);
#3711=FACE_OUTER_BOUND('',#4719,.T.);
#3712=FACE_OUTER_BOUND('',#4720,.T.);
#3713=FACE_OUTER_BOUND('',#4721,.T.);
#3714=FACE_OUTER_BOUND('',#4722,.T.);
#3715=FACE_OUTER_BOUND('',#4723,.T.);
#3716=FACE_OUTER_BOUND('',#4724,.T.);
#3717=FACE_OUTER_BOUND('',#4725,.T.);
#3718=FACE_OUTER_BOUND('',#4726,.T.);
#3719=FACE_OUTER_BOUND('',#4727,.T.);
#3720=FACE_OUTER_BOUND('',#4728,.T.);
#3721=FACE_OUTER_BOUND('',#4729,.T.);
#3722=FACE_OUTER_BOUND('',#4730,.T.);
#3723=FACE_OUTER_BOUND('',#4731,.T.);
#3724=FACE_OUTER_BOUND('',#4732,.T.);
#3725=FACE_OUTER_BOUND('',#4733,.T.);
#3726=FACE_OUTER_BOUND('',#4734,.T.);
#3727=FACE_OUTER_BOUND('',#4735,.T.);
#3728=FACE_OUTER_BOUND('',#4736,.T.);
#3729=FACE_OUTER_BOUND('',#4737,.T.);
#3730=FACE_OUTER_BOUND('',#4738,.T.);
#4550=EDGE_LOOP('',(#11069,#11070,#11071,#11072,#11073,#11074,#11075,#11076,
#11077,#11078,#11079,#11080,#11081,#11082,#11083,#11084,#11085,#11086,#11087,
#11088,#11089,#11090,#11091,#11092,#11093,#11094,#11095,#11096,#11097,#11098,
#11099,#11100,#11101,#11102,#11103,#11104,#11105,#11106,#11107,#11108,#11109,
#11110,#11111,#11112,#11113,#11114,#11115,#11116,#11117,#11118,#11119,#11120,
#11121,#11122,#11123,#11124,#11125,#11126,#11127,#11128,#11129,#11130,#11131,
#11132,#11133,#11134,#11135,#11136,#11137,#11138,#11139,#11140,#11141,#11142,
#11143,#11144,#11145,#11146,#11147,#11148,#11149,#11150,#11151,#11152,#11153,
#11154,#11155,#11156,#11157,#11158,#11159,#11160,#11161,#11162,#11163,#11164,
#11165,#11166,#11167,#11168,#11169,#11170,#11171,#11172,#11173,#11174,#11175,
#11176,#11177,#11178,#11179,#11180,#11181,#11182,#11183,#11184,#11185,#11186,
#11187,#11188,#11189,#11190,#11191,#11192,#11193,#11194,#11195,#11196,#11197,
#11198,#11199,#11200,#11201,#11202,#11203,#11204,#11205,#11206,#11207,#11208,
#11209,#11210,#11211,#11212,#11213,#11214,#11215,#11216,#11217,#11218,#11219,
#11220,#11221,#11222,#11223,#11224,#11225,#11226,#11227,#11228,#11229,#11230,
#11231,#11232,#11233,#11234,#11235,#11236,#11237,#11238,#11239,#11240,#11241,
#11242,#11243,#11244,#11245,#11246,#11247,#11248,#11249,#11250,#11251,#11252));
#4551=EDGE_LOOP('',(#11253));
#4552=EDGE_LOOP('',(#11254,#11255,#11256,#11257));
#4553=EDGE_LOOP('',(#11258,#11259,#11260,#11261));
#4554=EDGE_LOOP('',(#11262,#11263,#11264,#11265));
#4555=EDGE_LOOP('',(#11266,#11267,#11268,#11269));
#4556=EDGE_LOOP('',(#11270,#11271,#11272,#11273));
#4557=EDGE_LOOP('',(#11274,#11275,#11276,#11277));
#4558=EDGE_LOOP('',(#11278,#11279,#11280,#11281));
#4559=EDGE_LOOP('',(#11282,#11283,#11284,#11285));
#4560=EDGE_LOOP('',(#11286,#11287,#11288,#11289));
#4561=EDGE_LOOP('',(#11290,#11291,#11292,#11293));
#4562=EDGE_LOOP('',(#11294,#11295,#11296,#11297));
#4563=EDGE_LOOP('',(#11298,#11299,#11300,#11301));
#4564=EDGE_LOOP('',(#11302,#11303,#11304,#11305));
#4565=EDGE_LOOP('',(#11306,#11307,#11308,#11309));
#4566=EDGE_LOOP('',(#11310,#11311,#11312,#11313));
#4567=EDGE_LOOP('',(#11314,#11315,#11316,#11317));
#4568=EDGE_LOOP('',(#11318,#11319,#11320,#11321));
#4569=EDGE_LOOP('',(#11322,#11323,#11324,#11325));
#4570=EDGE_LOOP('',(#11326,#11327,#11328,#11329));
#4571=EDGE_LOOP('',(#11330,#11331,#11332,#11333));
#4572=EDGE_LOOP('',(#11334,#11335,#11336,#11337));
#4573=EDGE_LOOP('',(#11338,#11339,#11340,#11341));
#4574=EDGE_LOOP('',(#11342,#11343,#11344,#11345));
#4575=EDGE_LOOP('',(#11346,#11347,#11348,#11349));
#4576=EDGE_LOOP('',(#11350,#11351,#11352,#11353));
#4577=EDGE_LOOP('',(#11354,#11355,#11356,#11357));
#4578=EDGE_LOOP('',(#11358,#11359,#11360,#11361));
#4579=EDGE_LOOP('',(#11362,#11363,#11364,#11365));
#4580=EDGE_LOOP('',(#11366,#11367,#11368,#11369));
#4581=EDGE_LOOP('',(#11370,#11371,#11372,#11373));
#4582=EDGE_LOOP('',(#11374,#11375,#11376,#11377));
#4583=EDGE_LOOP('',(#11378,#11379,#11380,#11381));
#4584=EDGE_LOOP('',(#11382,#11383,#11384,#11385));
#4585=EDGE_LOOP('',(#11386,#11387,#11388,#11389));
#4586=EDGE_LOOP('',(#11390,#11391,#11392,#11393));
#4587=EDGE_LOOP('',(#11394,#11395,#11396,#11397));
#4588=EDGE_LOOP('',(#11398,#11399,#11400,#11401));
#4589=EDGE_LOOP('',(#11402,#11403,#11404,#11405));
#4590=EDGE_LOOP('',(#11406,#11407,#11408,#11409));
#4591=EDGE_LOOP('',(#11410,#11411,#11412,#11413));
#4592=EDGE_LOOP('',(#11414,#11415,#11416,#11417));
#4593=EDGE_LOOP('',(#11418,#11419,#11420,#11421));
#4594=EDGE_LOOP('',(#11422,#11423,#11424,#11425));
#4595=EDGE_LOOP('',(#11426,#11427,#11428,#11429));
#4596=EDGE_LOOP('',(#11430,#11431,#11432,#11433));
#4597=EDGE_LOOP('',(#11434,#11435,#11436,#11437,#11438,#11439,#11440,#11441,
#11442,#11443,#11444,#11445,#11446,#11447,#11448,#11449,#11450,#11451,#11452,
#11453,#11454,#11455,#11456,#11457,#11458,#11459,#11460,#11461,#11462,#11463,
#11464,#11465,#11466,#11467,#11468,#11469,#11470,#11471,#11472,#11473,#11474,
#11475,#11476,#11477,#11478,#11479,#11480,#11481,#11482,#11483,#11484,#11485,
#11486,#11487,#11488,#11489,#11490,#11491,#11492,#11493,#11494,#11495,#11496,
#11497,#11498,#11499,#11500,#11501,#11502,#11503,#11504,#11505,#11506,#11507,
#11508,#11509,#11510,#11511,#11512,#11513,#11514,#11515,#11516,#11517,#11518,
#11519,#11520,#11521,#11522,#11523,#11524,#11525,#11526,#11527,#11528,#11529,
#11530,#11531,#11532,#11533,#11534,#11535,#11536,#11537,#11538,#11539,#11540,
#11541,#11542,#11543,#11544,#11545,#11546,#11547,#11548,#11549,#11550,#11551,
#11552,#11553,#11554,#11555,#11556,#11557,#11558,#11559,#11560,#11561,#11562,
#11563,#11564,#11565,#11566,#11567,#11568,#11569,#11570,#11571,#11572,#11573,
#11574,#11575,#11576,#11577,#11578,#11579,#11580,#11581,#11582,#11583,#11584,
#11585,#11586,#11587,#11588,#11589,#11590,#11591,#11592,#11593,#11594,#11595,
#11596,#11597,#11598,#11599,#11600,#11601,#11602,#11603,#11604,#11605,#11606,
#11607,#11608,#11609,#11610,#11611,#11612,#11613,#11614,#11615,#11616,#11617));
#4598=EDGE_LOOP('',(#11618));
#4599=EDGE_LOOP('',(#11619,#11620,#11621,#11622));
#4600=EDGE_LOOP('',(#11623,#11624,#11625,#11626));
#4601=EDGE_LOOP('',(#11627,#11628,#11629,#11630));
#4602=EDGE_LOOP('',(#11631,#11632,#11633,#11634));
#4603=EDGE_LOOP('',(#11635,#11636,#11637,#11638));
#4604=EDGE_LOOP('',(#11639,#11640,#11641,#11642));
#4605=EDGE_LOOP('',(#11643,#11644,#11645,#11646));
#4606=EDGE_LOOP('',(#11647,#11648,#11649,#11650));
#4607=EDGE_LOOP('',(#11651,#11652,#11653,#11654));
#4608=EDGE_LOOP('',(#11655,#11656,#11657,#11658));
#4609=EDGE_LOOP('',(#11659,#11660,#11661,#11662));
#4610=EDGE_LOOP('',(#11663,#11664,#11665,#11666));
#4611=EDGE_LOOP('',(#11667,#11668,#11669,#11670));
#4612=EDGE_LOOP('',(#11671,#11672,#11673,#11674));
#4613=EDGE_LOOP('',(#11675,#11676,#11677,#11678));
#4614=EDGE_LOOP('',(#11679,#11680,#11681,#11682));
#4615=EDGE_LOOP('',(#11683,#11684,#11685,#11686));
#4616=EDGE_LOOP('',(#11687,#11688,#11689,#11690));
#4617=EDGE_LOOP('',(#11691,#11692,#11693,#11694));
#4618=EDGE_LOOP('',(#11695,#11696,#11697,#11698));
#4619=EDGE_LOOP('',(#11699,#11700,#11701,#11702));
#4620=EDGE_LOOP('',(#11703,#11704,#11705,#11706));
#4621=EDGE_LOOP('',(#11707,#11708,#11709,#11710));
#4622=EDGE_LOOP('',(#11711,#11712,#11713,#11714));
#4623=EDGE_LOOP('',(#11715,#11716,#11717,#11718));
#4624=EDGE_LOOP('',(#11719,#11720,#11721,#11722));
#4625=EDGE_LOOP('',(#11723,#11724,#11725,#11726));
#4626=EDGE_LOOP('',(#11727,#11728,#11729,#11730));
#4627=EDGE_LOOP('',(#11731,#11732,#11733,#11734));
#4628=EDGE_LOOP('',(#11735,#11736,#11737,#11738));
#4629=EDGE_LOOP('',(#11739,#11740,#11741,#11742));
#4630=EDGE_LOOP('',(#11743,#11744,#11745,#11746));
#4631=EDGE_LOOP('',(#11747,#11748,#11749,#11750));
#4632=EDGE_LOOP('',(#11751,#11752,#11753,#11754));
#4633=EDGE_LOOP('',(#11755,#11756,#11757,#11758));
#4634=EDGE_LOOP('',(#11759,#11760,#11761,#11762));
#4635=EDGE_LOOP('',(#11763,#11764,#11765,#11766));
#4636=EDGE_LOOP('',(#11767,#11768,#11769,#11770));
#4637=EDGE_LOOP('',(#11771,#11772,#11773,#11774));
#4638=EDGE_LOOP('',(#11775,#11776,#11777,#11778));
#4639=EDGE_LOOP('',(#11779,#11780,#11781,#11782));
#4640=EDGE_LOOP('',(#11783,#11784,#11785,#11786));
#4641=EDGE_LOOP('',(#11787,#11788,#11789,#11790));
#4642=EDGE_LOOP('',(#11791,#11792,#11793,#11794));
#4643=EDGE_LOOP('',(#11795,#11796,#11797,#11798));
#4644=EDGE_LOOP('',(#11799,#11800,#11801,#11802));
#4645=EDGE_LOOP('',(#11803,#11804,#11805,#11806));
#4646=EDGE_LOOP('',(#11807,#11808,#11809,#11810));
#4647=EDGE_LOOP('',(#11811,#11812,#11813,#11814));
#4648=EDGE_LOOP('',(#11815,#11816,#11817,#11818));
#4649=EDGE_LOOP('',(#11819,#11820,#11821,#11822));
#4650=EDGE_LOOP('',(#11823,#11824,#11825,#11826));
#4651=EDGE_LOOP('',(#11827,#11828,#11829,#11830));
#4652=EDGE_LOOP('',(#11831,#11832,#11833,#11834));
#4653=EDGE_LOOP('',(#11835,#11836,#11837,#11838));
#4654=EDGE_LOOP('',(#11839,#11840,#11841,#11842));
#4655=EDGE_LOOP('',(#11843,#11844,#11845,#11846));
#4656=EDGE_LOOP('',(#11847,#11848,#11849,#11850));
#4657=EDGE_LOOP('',(#11851,#11852,#11853,#11854));
#4658=EDGE_LOOP('',(#11855,#11856,#11857,#11858));
#4659=EDGE_LOOP('',(#11859,#11860,#11861,#11862));
#4660=EDGE_LOOP('',(#11863,#11864,#11865,#11866));
#4661=EDGE_LOOP('',(#11867,#11868,#11869,#11870));
#4662=EDGE_LOOP('',(#11871,#11872,#11873,#11874));
#4663=EDGE_LOOP('',(#11875,#11876,#11877,#11878));
#4664=EDGE_LOOP('',(#11879,#11880,#11881,#11882));
#4665=EDGE_LOOP('',(#11883,#11884,#11885,#11886));
#4666=EDGE_LOOP('',(#11887,#11888,#11889,#11890));
#4667=EDGE_LOOP('',(#11891,#11892,#11893,#11894));
#4668=EDGE_LOOP('',(#11895,#11896,#11897,#11898));
#4669=EDGE_LOOP('',(#11899,#11900,#11901,#11902));
#4670=EDGE_LOOP('',(#11903,#11904,#11905,#11906));
#4671=EDGE_LOOP('',(#11907,#11908,#11909,#11910));
#4672=EDGE_LOOP('',(#11911,#11912,#11913,#11914));
#4673=EDGE_LOOP('',(#11915,#11916,#11917,#11918));
#4674=EDGE_LOOP('',(#11919,#11920,#11921,#11922));
#4675=EDGE_LOOP('',(#11923,#11924,#11925,#11926));
#4676=EDGE_LOOP('',(#11927,#11928,#11929,#11930));
#4677=EDGE_LOOP('',(#11931,#11932,#11933,#11934));
#4678=EDGE_LOOP('',(#11935,#11936,#11937,#11938));
#4679=EDGE_LOOP('',(#11939,#11940,#11941,#11942));
#4680=EDGE_LOOP('',(#11943,#11944,#11945,#11946));
#4681=EDGE_LOOP('',(#11947,#11948,#11949,#11950));
#4682=EDGE_LOOP('',(#11951,#11952,#11953,#11954));
#4683=EDGE_LOOP('',(#11955,#11956,#11957,#11958));
#4684=EDGE_LOOP('',(#11959,#11960,#11961,#11962));
#4685=EDGE_LOOP('',(#11963,#11964,#11965,#11966));
#4686=EDGE_LOOP('',(#11967,#11968,#11969,#11970));
#4687=EDGE_LOOP('',(#11971,#11972,#11973,#11974));
#4688=EDGE_LOOP('',(#11975,#11976,#11977,#11978));
#4689=EDGE_LOOP('',(#11979,#11980,#11981,#11982));
#4690=EDGE_LOOP('',(#11983,#11984,#11985,#11986));
#4691=EDGE_LOOP('',(#11987,#11988,#11989,#11990));
#4692=EDGE_LOOP('',(#11991,#11992,#11993,#11994));
#4693=EDGE_LOOP('',(#11995,#11996,#11997,#11998));
#4694=EDGE_LOOP('',(#11999,#12000,#12001,#12002));
#4695=EDGE_LOOP('',(#12003,#12004,#12005,#12006));
#4696=EDGE_LOOP('',(#12007,#12008,#12009,#12010));
#4697=EDGE_LOOP('',(#12011,#12012,#12013,#12014));
#4698=EDGE_LOOP('',(#12015,#12016,#12017,#12018));
#4699=EDGE_LOOP('',(#12019,#12020,#12021,#12022));
#4700=EDGE_LOOP('',(#12023,#12024,#12025,#12026));
#4701=EDGE_LOOP('',(#12027,#12028,#12029,#12030));
#4702=EDGE_LOOP('',(#12031,#12032,#12033,#12034));
#4703=EDGE_LOOP('',(#12035,#12036,#12037,#12038));
#4704=EDGE_LOOP('',(#12039,#12040,#12041,#12042));
#4705=EDGE_LOOP('',(#12043,#12044,#12045,#12046));
#4706=EDGE_LOOP('',(#12047,#12048,#12049,#12050));
#4707=EDGE_LOOP('',(#12051,#12052,#12053,#12054));
#4708=EDGE_LOOP('',(#12055,#12056,#12057,#12058));
#4709=EDGE_LOOP('',(#12059,#12060,#12061,#12062));
#4710=EDGE_LOOP('',(#12063,#12064,#12065,#12066));
#4711=EDGE_LOOP('',(#12067,#12068,#12069,#12070));
#4712=EDGE_LOOP('',(#12071,#12072,#12073,#12074));
#4713=EDGE_LOOP('',(#12075,#12076,#12077,#12078));
#4714=EDGE_LOOP('',(#12079,#12080,#12081,#12082));
#4715=EDGE_LOOP('',(#12083,#12084,#12085,#12086));
#4716=EDGE_LOOP('',(#12087,#12088,#12089,#12090));
#4717=EDGE_LOOP('',(#12091,#12092,#12093,#12094));
#4718=EDGE_LOOP('',(#12095,#12096,#12097,#12098));
#4719=EDGE_LOOP('',(#12099,#12100,#12101,#12102));
#4720=EDGE_LOOP('',(#12103,#12104,#12105,#12106));
#4721=EDGE_LOOP('',(#12107,#12108,#12109,#12110));
#4722=EDGE_LOOP('',(#12111,#12112,#12113,#12114));
#4723=EDGE_LOOP('',(#12115,#12116,#12117,#12118));
#4724=EDGE_LOOP('',(#12119,#12120,#12121,#12122));
#4725=EDGE_LOOP('',(#12123,#12124,#12125,#12126));
#4726=EDGE_LOOP('',(#12127,#12128,#12129,#12130));
#4727=EDGE_LOOP('',(#12131,#12132,#12133,#12134));
#4728=EDGE_LOOP('',(#12135,#12136,#12137,#12138));
#4729=EDGE_LOOP('',(#12139,#12140,#12141,#12142));
#4730=EDGE_LOOP('',(#12143,#12144,#12145,#12146));
#4731=EDGE_LOOP('',(#12147,#12148,#12149,#12150));
#4732=EDGE_LOOP('',(#12151,#12152,#12153,#12154));
#4733=EDGE_LOOP('',(#12155,#12156,#12157,#12158));
#4734=EDGE_LOOP('',(#12159,#12160,#12161,#12162));
#4735=EDGE_LOOP('',(#12163,#12164,#12165,#12166));
#4736=EDGE_LOOP('',(#12167,#12168,#12169,#12170));
#4737=EDGE_LOOP('',(#12171,#12172,#12173,#12174));
#4738=EDGE_LOOP('',(#12175,#12176,#12177,#12178));
#5623=CIRCLE('',#17838,0.0046);
#5624=CIRCLE('',#17839,0.010874);
#5625=CIRCLE('',#17840,0.0046);
#5626=CIRCLE('',#17841,0.012);
#5627=CIRCLE('',#17842,0.0046);
#5628=CIRCLE('',#17843,0.010874);
#5629=CIRCLE('',#17844,0.0046);
#5630=CIRCLE('',#17845,0.012);
#5631=CIRCLE('',#17846,0.0046);
#5632=CIRCLE('',#17847,0.010874);
#5633=CIRCLE('',#17848,0.0046);
#5634=CIRCLE('',#17849,0.012);
#5635=CIRCLE('',#17850,0.0046);
#5636=CIRCLE('',#17851,0.010874);
#5637=CIRCLE('',#17852,0.0046);
#5638=CIRCLE('',#17853,0.012);
#5639=CIRCLE('',#17854,0.0046);
#5640=CIRCLE('',#17855,0.010874);
#5641=CIRCLE('',#17856,0.0046);
#5642=CIRCLE('',#17857,0.012);
#5643=CIRCLE('',#17858,0.0046);
#5644=CIRCLE('',#17859,0.010874);
#5645=CIRCLE('',#17860,0.0046);
#5646=CIRCLE('',#17861,0.012);
#5647=CIRCLE('',#17862,0.0046);
#5648=CIRCLE('',#17863,0.010874);
#5649=CIRCLE('',#17864,0.0046);
#5650=CIRCLE('',#17865,0.012);
#5651=CIRCLE('',#17866,0.0046);
#5652=CIRCLE('',#17867,0.010874);
#5653=CIRCLE('',#17868,0.0046);
#5654=CIRCLE('',#17869,0.012);
#5655=CIRCLE('',#17870,0.0046);
#5656=CIRCLE('',#17871,0.010874);
#5657=CIRCLE('',#17872,0.0046);
#5658=CIRCLE('',#17873,0.012);
#5659=CIRCLE('',#17874,0.0046);
#5660=CIRCLE('',#17875,0.010874);
#5661=CIRCLE('',#17876,0.0046);
#5662=CIRCLE('',#17877,0.012);
#5663=CIRCLE('',#17878,0.0046);
#5664=CIRCLE('',#17879,0.010874);
#5665=CIRCLE('',#17880,0.0046);
#5666=CIRCLE('',#17881,0.012);
#5667=CIRCLE('',#17882,0.0046);
#5668=CIRCLE('',#17883,0.010874);
#5669=CIRCLE('',#17884,0.0046);
#5670=CIRCLE('',#17885,0.012);
#5671=CIRCLE('',#17886,0.0046);
#5672=CIRCLE('',#17887,0.010874);
#5673=CIRCLE('',#17888,0.0046);
#5674=CIRCLE('',#17889,0.012);
#5675=CIRCLE('',#17890,0.0046);
#5676=CIRCLE('',#17891,0.010874);
#5677=CIRCLE('',#17892,0.0046);
#5678=CIRCLE('',#17893,0.012);
#5679=CIRCLE('',#17894,0.0046);
#5680=CIRCLE('',#17895,0.010874);
#5681=CIRCLE('',#17896,0.0046);
#5682=CIRCLE('',#17897,0.012);
#5683=CIRCLE('',#17898,0.0046);
#5684=CIRCLE('',#17899,0.010874);
#5685=CIRCLE('',#17900,0.0046);
#5686=CIRCLE('',#17901,0.012);
#5687=CIRCLE('',#17902,0.0046);
#5688=CIRCLE('',#17903,0.010874);
#5689=CIRCLE('',#17904,0.0046);
#5690=CIRCLE('',#17905,0.012);
#5691=CIRCLE('',#17906,0.0046);
#5692=CIRCLE('',#17907,0.010874);
#5693=CIRCLE('',#17908,0.0046);
#5694=CIRCLE('',#17909,0.012);
#5695=CIRCLE('',#17910,0.0046);
#5696=CIRCLE('',#17911,0.010874);
#5697=CIRCLE('',#17912,0.0046);
#5698=CIRCLE('',#17913,0.012);
#5699=CIRCLE('',#17914,0.0046);
#5700=CIRCLE('',#17915,0.010874);
#5701=CIRCLE('',#17916,0.0046);
#5702=CIRCLE('',#17917,0.012);
#5703=CIRCLE('',#17918,0.0046);
#5704=CIRCLE('',#17919,0.010874);
#5705=CIRCLE('',#17920,0.0046);
#5706=CIRCLE('',#17921,0.012);
#5707=CIRCLE('',#17922,0.0046);
#5708=CIRCLE('',#17923,0.010874);
#5709=CIRCLE('',#17924,0.0046);
#5710=CIRCLE('',#17925,0.012);
#5711=CIRCLE('',#17926,0.0046);
#5712=CIRCLE('',#17927,0.010874);
#5713=CIRCLE('',#17928,0.0046);
#5714=CIRCLE('',#17929,0.012);
#5715=CIRCLE('',#17930,0.0046);
#5716=CIRCLE('',#17931,0.010874);
#5717=CIRCLE('',#17932,0.0046);
#5718=CIRCLE('',#17933,0.012);
#5719=CIRCLE('',#17934,0.0046);
#5720=CIRCLE('',#17935,0.010874);
#5721=CIRCLE('',#17936,0.0046);
#5722=CIRCLE('',#17937,0.012);
#5723=CIRCLE('',#17938,0.0046);
#5724=CIRCLE('',#17939,0.010874);
#5725=CIRCLE('',#17940,0.0046);
#5726=CIRCLE('',#17941,0.012);
#5727=CIRCLE('',#17942,0.0046);
#5728=CIRCLE('',#17943,0.010874);
#5729=CIRCLE('',#17944,0.0046);
#5730=CIRCLE('',#17945,0.012);
#5731=CIRCLE('',#17946,0.0046);
#5732=CIRCLE('',#17947,0.010874);
#5733=CIRCLE('',#17948,0.0046);
#5734=CIRCLE('',#17949,0.012);
#5735=CIRCLE('',#17950,0.0046);
#5736=CIRCLE('',#17951,0.010874);
#5737=CIRCLE('',#17952,0.0046);
#5738=CIRCLE('',#17953,0.012);
#5739=CIRCLE('',#17954,0.0046);
#5740=CIRCLE('',#17955,0.010874);
#5741=CIRCLE('',#17956,0.0046);
#5742=CIRCLE('',#17957,0.012);
#5743=CIRCLE('',#17958,0.0046);
#5744=CIRCLE('',#17959,0.010874);
#5745=CIRCLE('',#17960,0.0046);
#5746=CIRCLE('',#17961,0.012);
#5747=CIRCLE('',#17962,0.0046);
#5748=CIRCLE('',#17963,0.010874);
#5749=CIRCLE('',#17964,0.0046);
#5750=CIRCLE('',#17965,0.012);
#5751=CIRCLE('',#17966,0.0046);
#5752=CIRCLE('',#17967,0.010874);
#5753=CIRCLE('',#17968,0.0046);
#5754=CIRCLE('',#17969,0.012);
#5755=CIRCLE('',#17970,0.0046);
#5756=CIRCLE('',#17971,0.010874);
#5757=CIRCLE('',#17972,0.0046);
#5758=CIRCLE('',#17973,0.012);
#5759=CIRCLE('',#17974,0.0046);
#5760=CIRCLE('',#17975,0.010874);
#5761=CIRCLE('',#17976,0.0046);
#5762=CIRCLE('',#17977,0.012);
#5763=CIRCLE('',#17978,0.0046);
#5764=CIRCLE('',#17979,0.010874);
#5765=CIRCLE('',#17980,0.0046);
#5766=CIRCLE('',#17981,0.012);
#5767=CIRCLE('',#17982,0.0046);
#5768=CIRCLE('',#17983,0.010874);
#5769=CIRCLE('',#17984,0.0046);
#5770=CIRCLE('',#17985,0.012);
#5771=CIRCLE('',#17986,0.0046);
#5772=CIRCLE('',#17987,0.010874);
#5773=CIRCLE('',#17988,0.0046);
#5774=CIRCLE('',#17989,0.012);
#5775=CIRCLE('',#17990,0.0046);
#5776=CIRCLE('',#17991,0.010874);
#5777=CIRCLE('',#17992,0.0046);
#5778=CIRCLE('',#17993,0.012);
#5779=CIRCLE('',#17994,0.0046);
#5780=CIRCLE('',#17995,0.010874);
#5781=CIRCLE('',#17996,0.0046);
#5782=CIRCLE('',#17997,0.012);
#5783=CIRCLE('',#17998,0.0046);
#5784=CIRCLE('',#17999,0.010874);
#5785=CIRCLE('',#18000,0.0046);
#5786=CIRCLE('',#18001,0.012);
#5787=CIRCLE('',#18002,0.0046);
#5788=CIRCLE('',#18003,0.010874);
#5789=CIRCLE('',#18004,0.0046);
#5790=CIRCLE('',#18005,0.012);
#5791=CIRCLE('',#18006,0.0046);
#5792=CIRCLE('',#18007,0.010874);
#5793=CIRCLE('',#18008,0.0046);
#5794=CIRCLE('',#18009,0.012);
#5795=CIRCLE('',#18010,0.0046);
#5796=CIRCLE('',#18011,0.010874);
#5797=CIRCLE('',#18012,0.0046);
#5798=CIRCLE('',#18013,0.012);
#5799=CIRCLE('',#18014,0.0046);
#5800=CIRCLE('',#18015,0.010874);
#5801=CIRCLE('',#18016,0.0046);
#5802=CIRCLE('',#18017,0.012);
#5803=CIRCLE('',#18018,0.0046);
#5804=CIRCLE('',#18019,0.010874);
#5805=CIRCLE('',#18020,0.0046);
#5806=CIRCLE('',#18021,0.012);
#5807=CIRCLE('',#18022,0.009);
#5808=CIRCLE('',#18024,0.012);
#5809=CIRCLE('',#18026,0.012);
#5810=CIRCLE('',#18028,0.012);
#5811=CIRCLE('',#18030,0.012);
#5812=CIRCLE('',#18032,0.012);
#5813=CIRCLE('',#18034,0.012);
#5814=CIRCLE('',#18036,0.012);
#5815=CIRCLE('',#18038,0.012);
#5816=CIRCLE('',#18040,0.012);
#5817=CIRCLE('',#18042,0.012);
#5818=CIRCLE('',#18044,0.012);
#5819=CIRCLE('',#18046,0.012);
#5820=CIRCLE('',#18048,0.012);
#5821=CIRCLE('',#18050,0.012);
#5822=CIRCLE('',#18052,0.012);
#5823=CIRCLE('',#18054,0.012);
#5824=CIRCLE('',#18056,0.012);
#5825=CIRCLE('',#18058,0.012);
#5826=CIRCLE('',#18060,0.012);
#5827=CIRCLE('',#18062,0.012);
#5828=CIRCLE('',#18064,0.012);
#5829=CIRCLE('',#18066,0.012);
#5830=CIRCLE('',#18068,0.012);
#5831=CIRCLE('',#18070,0.012);
#5832=CIRCLE('',#18072,0.012);
#5833=CIRCLE('',#18074,0.012);
#5834=CIRCLE('',#18076,0.012);
#5835=CIRCLE('',#18078,0.012);
#5836=CIRCLE('',#18080,0.012);
#5837=CIRCLE('',#18082,0.012);
#5838=CIRCLE('',#18084,0.012);
#5839=CIRCLE('',#18086,0.012);
#5840=CIRCLE('',#18088,0.012);
#5841=CIRCLE('',#18090,0.012);
#5842=CIRCLE('',#18092,0.012);
#5843=CIRCLE('',#18094,0.012);
#5844=CIRCLE('',#18096,0.012);
#5845=CIRCLE('',#18098,0.012);
#5846=CIRCLE('',#18100,0.012);
#5847=CIRCLE('',#18102,0.012);
#5848=CIRCLE('',#18104,0.012);
#5849=CIRCLE('',#18106,0.012);
#5850=CIRCLE('',#18108,0.012);
#5851=CIRCLE('',#18110,0.012);
#5852=CIRCLE('',#18112,0.012);
#5853=CIRCLE('',#18114,0.0046);
#5854=CIRCLE('',#18115,0.0046);
#5855=CIRCLE('',#18116,0.010874);
#5856=CIRCLE('',#18117,0.0046);
#5857=CIRCLE('',#18118,0.0046);
#5858=CIRCLE('',#18119,0.010874);
#5859=CIRCLE('',#18120,0.0046);
#5860=CIRCLE('',#18121,0.0046);
#5861=CIRCLE('',#18122,0.010874);
#5862=CIRCLE('',#18123,0.0046);
#5863=CIRCLE('',#18124,0.0046);
#5864=CIRCLE('',#18125,0.010874);
#5865=CIRCLE('',#18126,0.0046);
#5866=CIRCLE('',#18127,0.0046);
#5867=CIRCLE('',#18128,0.010874);
#5868=CIRCLE('',#18129,0.0046);
#5869=CIRCLE('',#18130,0.0046);
#5870=CIRCLE('',#18131,0.010874);
#5871=CIRCLE('',#18132,0.0046);
#5872=CIRCLE('',#18133,0.0046);
#5873=CIRCLE('',#18134,0.010874);
#5874=CIRCLE('',#18135,0.0046);
#5875=CIRCLE('',#18136,0.0046);
#5876=CIRCLE('',#18137,0.010874);
#5877=CIRCLE('',#18138,0.0046);
#5878=CIRCLE('',#18139,0.0046);
#5879=CIRCLE('',#18140,0.010874);
#5880=CIRCLE('',#18141,0.0046);
#5881=CIRCLE('',#18142,0.0046);
#5882=CIRCLE('',#18143,0.010874);
#5883=CIRCLE('',#18144,0.0046);
#5884=CIRCLE('',#18145,0.0046);
#5885=CIRCLE('',#18146,0.010874);
#5886=CIRCLE('',#18147,0.0046);
#5887=CIRCLE('',#18148,0.012);
#5888=CIRCLE('',#18149,0.0046);
#5889=CIRCLE('',#18150,0.010874);
#5890=CIRCLE('',#18151,0.0046);
#5891=CIRCLE('',#18152,0.0046);
#5892=CIRCLE('',#18153,0.010874);
#5893=CIRCLE('',#18154,0.0046);
#5894=CIRCLE('',#18155,0.0046);
#5895=CIRCLE('',#18156,0.010874);
#5896=CIRCLE('',#18157,0.0046);
#5897=CIRCLE('',#18158,0.0046);
#5898=CIRCLE('',#18159,0.010874);
#5899=CIRCLE('',#18160,0.0046);
#5900=CIRCLE('',#18161,0.0046);
#5901=CIRCLE('',#18162,0.010874);
#5902=CIRCLE('',#18163,0.0046);
#5903=CIRCLE('',#18164,0.0046);
#5904=CIRCLE('',#18165,0.010874);
#5905=CIRCLE('',#18166,0.0046);
#5906=CIRCLE('',#18167,0.0046);
#5907=CIRCLE('',#18168,0.010874);
#5908=CIRCLE('',#18169,0.0046);
#5909=CIRCLE('',#18170,0.0046);
#5910=CIRCLE('',#18171,0.010874);
#5911=CIRCLE('',#18172,0.0046);
#5912=CIRCLE('',#18173,0.0046);
#5913=CIRCLE('',#18174,0.010874);
#5914=CIRCLE('',#18175,0.0046);
#5915=CIRCLE('',#18176,0.0046);
#5916=CIRCLE('',#18177,0.010874);
#5917=CIRCLE('',#18178,0.0046);
#5918=CIRCLE('',#18179,0.0046);
#5919=CIRCLE('',#18180,0.010874);
#5920=CIRCLE('',#18181,0.0046);
#5921=CIRCLE('',#18182,0.0046);
#5922=CIRCLE('',#18183,0.010874);
#5923=CIRCLE('',#18184,0.0046);
#5924=CIRCLE('',#18185,0.0046);
#5925=CIRCLE('',#18186,0.010874);
#5926=CIRCLE('',#18187,0.0046);
#5927=CIRCLE('',#18188,0.0046);
#5928=CIRCLE('',#18189,0.010874);
#5929=CIRCLE('',#18190,0.0046);
#5930=CIRCLE('',#18191,0.0046);
#5931=CIRCLE('',#18192,0.010874);
#5932=CIRCLE('',#18193,0.0046);
#5933=CIRCLE('',#18194,0.0046);
#5934=CIRCLE('',#18195,0.010874);
#5935=CIRCLE('',#18196,0.0046);
#5936=CIRCLE('',#18197,0.0046);
#5937=CIRCLE('',#18198,0.010874);
#5938=CIRCLE('',#18199,0.0046);
#5939=CIRCLE('',#18200,0.0046);
#5940=CIRCLE('',#18201,0.010874);
#5941=CIRCLE('',#18202,0.0046);
#5942=CIRCLE('',#18203,0.0046);
#5943=CIRCLE('',#18204,0.010874);
#5944=CIRCLE('',#18205,0.0046);
#5945=CIRCLE('',#18206,0.0046);
#5946=CIRCLE('',#18207,0.010874);
#5947=CIRCLE('',#18208,0.0046);
#5948=CIRCLE('',#18209,0.0046);
#5949=CIRCLE('',#18210,0.010874);
#5950=CIRCLE('',#18211,0.0046);
#5951=CIRCLE('',#18212,0.0046);
#5952=CIRCLE('',#18213,0.010874);
#5953=CIRCLE('',#18214,0.0046);
#5954=CIRCLE('',#18215,0.0046);
#5955=CIRCLE('',#18216,0.010874);
#5956=CIRCLE('',#18217,0.0046);
#5957=CIRCLE('',#18218,0.0046);
#5958=CIRCLE('',#18219,0.010874);
#5959=CIRCLE('',#18220,0.0046);
#5960=CIRCLE('',#18221,0.0046);
#5961=CIRCLE('',#18222,0.010874);
#5962=CIRCLE('',#18223,0.0046);
#5963=CIRCLE('',#18224,0.0046);
#5964=CIRCLE('',#18225,0.010874);
#5965=CIRCLE('',#18226,0.0046);
#5966=CIRCLE('',#18227,0.0046);
#5967=CIRCLE('',#18228,0.010874);
#5968=CIRCLE('',#18229,0.0046);
#5969=CIRCLE('',#18230,0.0046);
#5970=CIRCLE('',#18231,0.010874);
#5971=CIRCLE('',#18232,0.0046);
#5972=CIRCLE('',#18233,0.0046);
#5973=CIRCLE('',#18234,0.010874);
#5974=CIRCLE('',#18235,0.0046);
#5975=CIRCLE('',#18236,0.0046);
#5976=CIRCLE('',#18237,0.010874);
#5977=CIRCLE('',#18238,0.0046);
#5978=CIRCLE('',#18239,0.0046);
#5979=CIRCLE('',#18240,0.010874);
#5980=CIRCLE('',#18241,0.0046);
#5981=CIRCLE('',#18242,0.0046);
#5982=CIRCLE('',#18243,0.010874);
#5983=CIRCLE('',#18244,0.0046);
#5984=CIRCLE('',#18245,0.0046);
#5985=CIRCLE('',#18246,0.010874);
#5986=CIRCLE('',#18247,0.0046);
#5987=CIRCLE('',#18248,0.0046);
#5988=CIRCLE('',#18249,0.010874);
#5989=CIRCLE('',#18250,0.0046);
#5990=CIRCLE('',#18251,0.0046);
#5991=CIRCLE('',#18252,0.010874);
#5992=CIRCLE('',#18253,0.009);
#6526=VERTEX_POINT('',#23729);
#6527=VERTEX_POINT('',#23730);
#6528=VERTEX_POINT('',#23732);
#6529=VERTEX_POINT('',#23734);
#6530=VERTEX_POINT('',#23736);
#6531=VERTEX_POINT('',#23738);
#6532=VERTEX_POINT('',#23740);
#6533=VERTEX_POINT('',#23742);
#6534=VERTEX_POINT('',#23744);
#6535=VERTEX_POINT('',#23746);
#6536=VERTEX_POINT('',#23748);
#6537=VERTEX_POINT('',#23750);
#6538=VERTEX_POINT('',#23752);
#6539=VERTEX_POINT('',#23754);
#6540=VERTEX_POINT('',#23756);
#6541=VERTEX_POINT('',#23758);
#6542=VERTEX_POINT('',#23760);
#6543=VERTEX_POINT('',#23762);
#6544=VERTEX_POINT('',#23764);
#6545=VERTEX_POINT('',#23766);
#6546=VERTEX_POINT('',#23768);
#6547=VERTEX_POINT('',#23770);
#6548=VERTEX_POINT('',#23772);
#6549=VERTEX_POINT('',#23774);
#6550=VERTEX_POINT('',#23776);
#6551=VERTEX_POINT('',#23778);
#6552=VERTEX_POINT('',#23780);
#6553=VERTEX_POINT('',#23782);
#6554=VERTEX_POINT('',#23784);
#6555=VERTEX_POINT('',#23786);
#6556=VERTEX_POINT('',#23788);
#6557=VERTEX_POINT('',#23790);
#6558=VERTEX_POINT('',#23792);
#6559=VERTEX_POINT('',#23794);
#6560=VERTEX_POINT('',#23796);
#6561=VERTEX_POINT('',#23798);
#6562=VERTEX_POINT('',#23800);
#6563=VERTEX_POINT('',#23802);
#6564=VERTEX_POINT('',#23804);
#6565=VERTEX_POINT('',#23806);
#6566=VERTEX_POINT('',#23808);
#6567=VERTEX_POINT('',#23810);
#6568=VERTEX_POINT('',#23812);
#6569=VERTEX_POINT('',#23814);
#6570=VERTEX_POINT('',#23816);
#6571=VERTEX_POINT('',#23818);
#6572=VERTEX_POINT('',#23820);
#6573=VERTEX_POINT('',#23822);
#6574=VERTEX_POINT('',#23824);
#6575=VERTEX_POINT('',#23826);
#6576=VERTEX_POINT('',#23828);
#6577=VERTEX_POINT('',#23830);
#6578=VERTEX_POINT('',#23832);
#6579=VERTEX_POINT('',#23834);
#6580=VERTEX_POINT('',#23836);
#6581=VERTEX_POINT('',#23838);
#6582=VERTEX_POINT('',#23840);
#6583=VERTEX_POINT('',#23842);
#6584=VERTEX_POINT('',#23844);
#6585=VERTEX_POINT('',#23846);
#6586=VERTEX_POINT('',#23848);
#6587=VERTEX_POINT('',#23850);
#6588=VERTEX_POINT('',#23852);
#6589=VERTEX_POINT('',#23854);
#6590=VERTEX_POINT('',#23856);
#6591=VERTEX_POINT('',#23858);
#6592=VERTEX_POINT('',#23860);
#6593=VERTEX_POINT('',#23862);
#6594=VERTEX_POINT('',#23864);
#6595=VERTEX_POINT('',#23866);
#6596=VERTEX_POINT('',#23868);
#6597=VERTEX_POINT('',#23870);
#6598=VERTEX_POINT('',#23872);
#6599=VERTEX_POINT('',#23874);
#6600=VERTEX_POINT('',#23876);
#6601=VERTEX_POINT('',#23878);
#6602=VERTEX_POINT('',#23880);
#6603=VERTEX_POINT('',#23882);
#6604=VERTEX_POINT('',#23884);
#6605=VERTEX_POINT('',#23886);
#6606=VERTEX_POINT('',#23888);
#6607=VERTEX_POINT('',#23890);
#6608=VERTEX_POINT('',#23892);
#6609=VERTEX_POINT('',#23894);
#6610=VERTEX_POINT('',#23896);
#6611=VERTEX_POINT('',#23898);
#6612=VERTEX_POINT('',#23900);
#6613=VERTEX_POINT('',#23902);
#6614=VERTEX_POINT('',#23904);
#6615=VERTEX_POINT('',#23906);
#6616=VERTEX_POINT('',#23908);
#6617=VERTEX_POINT('',#23910);
#6618=VERTEX_POINT('',#23912);
#6619=VERTEX_POINT('',#23914);
#6620=VERTEX_POINT('',#23916);
#6621=VERTEX_POINT('',#23918);
#6622=VERTEX_POINT('',#23920);
#6623=VERTEX_POINT('',#23922);
#6624=VERTEX_POINT('',#23924);
#6625=VERTEX_POINT('',#23926);
#6626=VERTEX_POINT('',#23928);
#6627=VERTEX_POINT('',#23930);
#6628=VERTEX_POINT('',#23932);
#6629=VERTEX_POINT('',#23934);
#6630=VERTEX_POINT('',#23936);
#6631=VERTEX_POINT('',#23938);
#6632=VERTEX_POINT('',#23940);
#6633=VERTEX_POINT('',#23942);
#6634=VERTEX_POINT('',#23944);
#6635=VERTEX_POINT('',#23946);
#6636=VERTEX_POINT('',#23948);
#6637=VERTEX_POINT('',#23950);
#6638=VERTEX_POINT('',#23952);
#6639=VERTEX_POINT('',#23954);
#6640=VERTEX_POINT('',#23956);
#6641=VERTEX_POINT('',#23958);
#6642=VERTEX_POINT('',#23960);
#6643=VERTEX_POINT('',#23962);
#6644=VERTEX_POINT('',#23964);
#6645=VERTEX_POINT('',#23966);
#6646=VERTEX_POINT('',#23968);
#6647=VERTEX_POINT('',#23970);
#6648=VERTEX_POINT('',#23972);
#6649=VERTEX_POINT('',#23974);
#6650=VERTEX_POINT('',#23976);
#6651=VERTEX_POINT('',#23978);
#6652=VERTEX_POINT('',#23980);
#6653=VERTEX_POINT('',#23982);
#6654=VERTEX_POINT('',#23984);
#6655=VERTEX_POINT('',#23986);
#6656=VERTEX_POINT('',#23988);
#6657=VERTEX_POINT('',#23990);
#6658=VERTEX_POINT('',#23992);
#6659=VERTEX_POINT('',#23994);
#6660=VERTEX_POINT('',#23996);
#6661=VERTEX_POINT('',#23998);
#6662=VERTEX_POINT('',#24000);
#6663=VERTEX_POINT('',#24002);
#6664=VERTEX_POINT('',#24004);
#6665=VERTEX_POINT('',#24006);
#6666=VERTEX_POINT('',#24008);
#6667=VERTEX_POINT('',#24010);
#6668=VERTEX_POINT('',#24012);
#6669=VERTEX_POINT('',#24014);
#6670=VERTEX_POINT('',#24016);
#6671=VERTEX_POINT('',#24018);
#6672=VERTEX_POINT('',#24020);
#6673=VERTEX_POINT('',#24022);
#6674=VERTEX_POINT('',#24024);
#6675=VERTEX_POINT('',#24026);
#6676=VERTEX_POINT('',#24028);
#6677=VERTEX_POINT('',#24030);
#6678=VERTEX_POINT('',#24032);
#6679=VERTEX_POINT('',#24034);
#6680=VERTEX_POINT('',#24036);
#6681=VERTEX_POINT('',#24038);
#6682=VERTEX_POINT('',#24040);
#6683=VERTEX_POINT('',#24042);
#6684=VERTEX_POINT('',#24044);
#6685=VERTEX_POINT('',#24046);
#6686=VERTEX_POINT('',#24048);
#6687=VERTEX_POINT('',#24050);
#6688=VERTEX_POINT('',#24052);
#6689=VERTEX_POINT('',#24054);
#6690=VERTEX_POINT('',#24056);
#6691=VERTEX_POINT('',#24058);
#6692=VERTEX_POINT('',#24060);
#6693=VERTEX_POINT('',#24062);
#6694=VERTEX_POINT('',#24064);
#6695=VERTEX_POINT('',#24066);
#6696=VERTEX_POINT('',#24068);
#6697=VERTEX_POINT('',#24070);
#6698=VERTEX_POINT('',#24072);
#6699=VERTEX_POINT('',#24074);
#6700=VERTEX_POINT('',#24076);
#6701=VERTEX_POINT('',#24078);
#6702=VERTEX_POINT('',#24080);
#6703=VERTEX_POINT('',#24082);
#6704=VERTEX_POINT('',#24084);
#6705=VERTEX_POINT('',#24086);
#6706=VERTEX_POINT('',#24088);
#6707=VERTEX_POINT('',#24090);
#6708=VERTEX_POINT('',#24092);
#6709=VERTEX_POINT('',#24094);
#6710=VERTEX_POINT('',#24097);
#6711=VERTEX_POINT('',#24100);
#6712=VERTEX_POINT('',#24102);
#6713=VERTEX_POINT('',#24106);
#6714=VERTEX_POINT('',#24108);
#6715=VERTEX_POINT('',#24112);
#6716=VERTEX_POINT('',#24114);
#6717=VERTEX_POINT('',#24118);
#6718=VERTEX_POINT('',#24120);
#6719=VERTEX_POINT('',#24124);
#6720=VERTEX_POINT('',#24126);
#6721=VERTEX_POINT('',#24130);
#6722=VERTEX_POINT('',#24132);
#6723=VERTEX_POINT('',#24136);
#6724=VERTEX_POINT('',#24138);
#6725=VERTEX_POINT('',#24142);
#6726=VERTEX_POINT('',#24144);
#6727=VERTEX_POINT('',#24148);
#6728=VERTEX_POINT('',#24150);
#6729=VERTEX_POINT('',#24154);
#6730=VERTEX_POINT('',#24156);
#6731=VERTEX_POINT('',#24160);
#6732=VERTEX_POINT('',#24162);
#6733=VERTEX_POINT('',#24166);
#6734=VERTEX_POINT('',#24168);
#6735=VERTEX_POINT('',#24172);
#6736=VERTEX_POINT('',#24174);
#6737=VERTEX_POINT('',#24178);
#6738=VERTEX_POINT('',#24180);
#6739=VERTEX_POINT('',#24184);
#6740=VERTEX_POINT('',#24186);
#6741=VERTEX_POINT('',#24190);
#6742=VERTEX_POINT('',#24192);
#6743=VERTEX_POINT('',#24196);
#6744=VERTEX_POINT('',#24198);
#6745=VERTEX_POINT('',#24202);
#6746=VERTEX_POINT('',#24204);
#6747=VERTEX_POINT('',#24208);
#6748=VERTEX_POINT('',#24210);
#6749=VERTEX_POINT('',#24214);
#6750=VERTEX_POINT('',#24216);
#6751=VERTEX_POINT('',#24220);
#6752=VERTEX_POINT('',#24222);
#6753=VERTEX_POINT('',#24226);
#6754=VERTEX_POINT('',#24228);
#6755=VERTEX_POINT('',#24232);
#6756=VERTEX_POINT('',#24234);
#6757=VERTEX_POINT('',#24238);
#6758=VERTEX_POINT('',#24240);
#6759=VERTEX_POINT('',#24244);
#6760=VERTEX_POINT('',#24246);
#6761=VERTEX_POINT('',#24250);
#6762=VERTEX_POINT('',#24252);
#6763=VERTEX_POINT('',#24256);
#6764=VERTEX_POINT('',#24258);
#6765=VERTEX_POINT('',#24262);
#6766=VERTEX_POINT('',#24264);
#6767=VERTEX_POINT('',#24268);
#6768=VERTEX_POINT('',#24270);
#6769=VERTEX_POINT('',#24274);
#6770=VERTEX_POINT('',#24276);
#6771=VERTEX_POINT('',#24280);
#6772=VERTEX_POINT('',#24282);
#6773=VERTEX_POINT('',#24286);
#6774=VERTEX_POINT('',#24288);
#6775=VERTEX_POINT('',#24292);
#6776=VERTEX_POINT('',#24294);
#6777=VERTEX_POINT('',#24298);
#6778=VERTEX_POINT('',#24300);
#6779=VERTEX_POINT('',#24304);
#6780=VERTEX_POINT('',#24306);
#6781=VERTEX_POINT('',#24310);
#6782=VERTEX_POINT('',#24312);
#6783=VERTEX_POINT('',#24316);
#6784=VERTEX_POINT('',#24318);
#6785=VERTEX_POINT('',#24322);
#6786=VERTEX_POINT('',#24324);
#6787=VERTEX_POINT('',#24328);
#6788=VERTEX_POINT('',#24330);
#6789=VERTEX_POINT('',#24334);
#6790=VERTEX_POINT('',#24336);
#6791=VERTEX_POINT('',#24340);
#6792=VERTEX_POINT('',#24342);
#6793=VERTEX_POINT('',#24346);
#6794=VERTEX_POINT('',#24348);
#6795=VERTEX_POINT('',#24352);
#6796=VERTEX_POINT('',#24354);
#6797=VERTEX_POINT('',#24358);
#6798=VERTEX_POINT('',#24360);
#6799=VERTEX_POINT('',#24364);
#6800=VERTEX_POINT('',#24366);
#6801=VERTEX_POINT('',#24370);
#6802=VERTEX_POINT('',#24372);
#6803=VERTEX_POINT('',#24374);
#6804=VERTEX_POINT('',#24377);
#6805=VERTEX_POINT('',#24379);
#6806=VERTEX_POINT('',#24382);
#6807=VERTEX_POINT('',#24384);
#6808=VERTEX_POINT('',#24387);
#6809=VERTEX_POINT('',#24389);
#6810=VERTEX_POINT('',#24392);
#6811=VERTEX_POINT('',#24394);
#6812=VERTEX_POINT('',#24397);
#6813=VERTEX_POINT('',#24399);
#6814=VERTEX_POINT('',#24402);
#6815=VERTEX_POINT('',#24404);
#6816=VERTEX_POINT('',#24407);
#6817=VERTEX_POINT('',#24409);
#6818=VERTEX_POINT('',#24412);
#6819=VERTEX_POINT('',#24414);
#6820=VERTEX_POINT('',#24417);
#6821=VERTEX_POINT('',#24419);
#6822=VERTEX_POINT('',#24422);
#6823=VERTEX_POINT('',#24424);
#6824=VERTEX_POINT('',#24426);
#6825=VERTEX_POINT('',#24428);
#6826=VERTEX_POINT('',#24430);
#6827=VERTEX_POINT('',#24432);
#6828=VERTEX_POINT('',#24435);
#6829=VERTEX_POINT('',#24437);
#6830=VERTEX_POINT('',#24440);
#6831=VERTEX_POINT('',#24442);
#6832=VERTEX_POINT('',#24445);
#6833=VERTEX_POINT('',#24447);
#6834=VERTEX_POINT('',#24450);
#6835=VERTEX_POINT('',#24452);
#6836=VERTEX_POINT('',#24455);
#6837=VERTEX_POINT('',#24457);
#6838=VERTEX_POINT('',#24460);
#6839=VERTEX_POINT('',#24462);
#6840=VERTEX_POINT('',#24465);
#6841=VERTEX_POINT('',#24467);
#6842=VERTEX_POINT('',#24470);
#6843=VERTEX_POINT('',#24472);
#6844=VERTEX_POINT('',#24475);
#6845=VERTEX_POINT('',#24477);
#6846=VERTEX_POINT('',#24480);
#6847=VERTEX_POINT('',#24482);
#6848=VERTEX_POINT('',#24485);
#6849=VERTEX_POINT('',#24487);
#6850=VERTEX_POINT('',#24490);
#6851=VERTEX_POINT('',#24492);
#6852=VERTEX_POINT('',#24495);
#6853=VERTEX_POINT('',#24497);
#6854=VERTEX_POINT('',#24500);
#6855=VERTEX_POINT('',#24502);
#6856=VERTEX_POINT('',#24505);
#6857=VERTEX_POINT('',#24507);
#6858=VERTEX_POINT('',#24510);
#6859=VERTEX_POINT('',#24512);
#6860=VERTEX_POINT('',#24515);
#6861=VERTEX_POINT('',#24517);
#6862=VERTEX_POINT('',#24520);
#6863=VERTEX_POINT('',#24522);
#6864=VERTEX_POINT('',#24525);
#6865=VERTEX_POINT('',#24527);
#6866=VERTEX_POINT('',#24530);
#6867=VERTEX_POINT('',#24532);
#6868=VERTEX_POINT('',#24535);
#6869=VERTEX_POINT('',#24537);
#6870=VERTEX_POINT('',#24540);
#6871=VERTEX_POINT('',#24542);
#6872=VERTEX_POINT('',#24545);
#6873=VERTEX_POINT('',#24547);
#6874=VERTEX_POINT('',#24550);
#6875=VERTEX_POINT('',#24552);
#6876=VERTEX_POINT('',#24555);
#6877=VERTEX_POINT('',#24557);
#6878=VERTEX_POINT('',#24560);
#6879=VERTEX_POINT('',#24562);
#6880=VERTEX_POINT('',#24565);
#6881=VERTEX_POINT('',#24567);
#6882=VERTEX_POINT('',#24570);
#6883=VERTEX_POINT('',#24572);
#6884=VERTEX_POINT('',#24575);
#6885=VERTEX_POINT('',#24577);
#6886=VERTEX_POINT('',#24580);
#6887=VERTEX_POINT('',#24582);
#6888=VERTEX_POINT('',#24585);
#6889=VERTEX_POINT('',#24587);
#6890=VERTEX_POINT('',#24590);
#6891=VERTEX_POINT('',#24592);
#6892=VERTEX_POINT('',#24595);
#6893=VERTEX_POINT('',#24597);
#6894=VERTEX_POINT('',#24600);
#6895=VERTEX_POINT('',#24603);
#8326=EDGE_CURVE('',#6526,#6527,#5623,.T.);
#8327=EDGE_CURVE('',#6528,#6526,#5624,.T.);
#8328=EDGE_CURVE('',#6529,#6528,#5625,.T.);
#8329=EDGE_CURVE('',#6530,#6529,#5626,.T.);
#8330=EDGE_CURVE('',#6531,#6530,#5627,.T.);
#8331=EDGE_CURVE('',#6532,#6531,#5628,.T.);
#8332=EDGE_CURVE('',#6533,#6532,#5629,.T.);
#8333=EDGE_CURVE('',#6534,#6533,#5630,.T.);
#8334=EDGE_CURVE('',#6535,#6534,#5631,.T.);
#8335=EDGE_CURVE('',#6536,#6535,#5632,.T.);
#8336=EDGE_CURVE('',#6537,#6536,#5633,.T.);
#8337=EDGE_CURVE('',#6538,#6537,#5634,.T.);
#8338=EDGE_CURVE('',#6539,#6538,#5635,.T.);
#8339=EDGE_CURVE('',#6540,#6539,#5636,.T.);
#8340=EDGE_CURVE('',#6541,#6540,#5637,.T.);
#8341=EDGE_CURVE('',#6542,#6541,#5638,.T.);
#8342=EDGE_CURVE('',#6543,#6542,#5639,.T.);
#8343=EDGE_CURVE('',#6544,#6543,#5640,.T.);
#8344=EDGE_CURVE('',#6545,#6544,#5641,.T.);
#8345=EDGE_CURVE('',#6546,#6545,#5642,.T.);
#8346=EDGE_CURVE('',#6547,#6546,#5643,.T.);
#8347=EDGE_CURVE('',#6548,#6547,#5644,.T.);
#8348=EDGE_CURVE('',#6549,#6548,#5645,.T.);
#8349=EDGE_CURVE('',#6550,#6549,#5646,.T.);
#8350=EDGE_CURVE('',#6551,#6550,#5647,.T.);
#8351=EDGE_CURVE('',#6552,#6551,#5648,.T.);
#8352=EDGE_CURVE('',#6553,#6552,#5649,.T.);
#8353=EDGE_CURVE('',#6554,#6553,#5650,.T.);
#8354=EDGE_CURVE('',#6555,#6554,#5651,.T.);
#8355=EDGE_CURVE('',#6556,#6555,#5652,.T.);
#8356=EDGE_CURVE('',#6557,#6556,#5653,.T.);
#8357=EDGE_CURVE('',#6558,#6557,#5654,.T.);
#8358=EDGE_CURVE('',#6559,#6558,#5655,.T.);
#8359=EDGE_CURVE('',#6560,#6559,#5656,.T.);
#8360=EDGE_CURVE('',#6561,#6560,#5657,.T.);
#8361=EDGE_CURVE('',#6562,#6561,#5658,.T.);
#8362=EDGE_CURVE('',#6563,#6562,#5659,.T.);
#8363=EDGE_CURVE('',#6564,#6563,#5660,.T.);
#8364=EDGE_CURVE('',#6565,#6564,#5661,.T.);
#8365=EDGE_CURVE('',#6566,#6565,#5662,.T.);
#8366=EDGE_CURVE('',#6567,#6566,#5663,.T.);
#8367=EDGE_CURVE('',#6568,#6567,#5664,.T.);
#8368=EDGE_CURVE('',#6569,#6568,#5665,.T.);
#8369=EDGE_CURVE('',#6570,#6569,#5666,.T.);
#8370=EDGE_CURVE('',#6571,#6570,#5667,.T.);
#8371=EDGE_CURVE('',#6572,#6571,#5668,.T.);
#8372=EDGE_CURVE('',#6573,#6572,#5669,.T.);
#8373=EDGE_CURVE('',#6574,#6573,#5670,.T.);
#8374=EDGE_CURVE('',#6575,#6574,#5671,.T.);
#8375=EDGE_CURVE('',#6576,#6575,#5672,.T.);
#8376=EDGE_CURVE('',#6577,#6576,#5673,.T.);
#8377=EDGE_CURVE('',#6578,#6577,#5674,.T.);
#8378=EDGE_CURVE('',#6579,#6578,#5675,.T.);
#8379=EDGE_CURVE('',#6580,#6579,#5676,.T.);
#8380=EDGE_CURVE('',#6581,#6580,#5677,.T.);
#8381=EDGE_CURVE('',#6582,#6581,#5678,.T.);
#8382=EDGE_CURVE('',#6583,#6582,#5679,.T.);
#8383=EDGE_CURVE('',#6584,#6583,#5680,.T.);
#8384=EDGE_CURVE('',#6585,#6584,#5681,.T.);
#8385=EDGE_CURVE('',#6586,#6585,#5682,.T.);
#8386=EDGE_CURVE('',#6587,#6586,#5683,.T.);
#8387=EDGE_CURVE('',#6588,#6587,#5684,.T.);
#8388=EDGE_CURVE('',#6589,#6588,#5685,.T.);
#8389=EDGE_CURVE('',#6590,#6589,#5686,.T.);
#8390=EDGE_CURVE('',#6591,#6590,#5687,.T.);
#8391=EDGE_CURVE('',#6592,#6591,#5688,.T.);
#8392=EDGE_CURVE('',#6593,#6592,#5689,.T.);
#8393=EDGE_CURVE('',#6594,#6593,#5690,.T.);
#8394=EDGE_CURVE('',#6595,#6594,#5691,.T.);
#8395=EDGE_CURVE('',#6596,#6595,#5692,.T.);
#8396=EDGE_CURVE('',#6597,#6596,#5693,.T.);
#8397=EDGE_CURVE('',#6598,#6597,#5694,.T.);
#8398=EDGE_CURVE('',#6599,#6598,#5695,.T.);
#8399=EDGE_CURVE('',#6600,#6599,#5696,.T.);
#8400=EDGE_CURVE('',#6601,#6600,#5697,.T.);
#8401=EDGE_CURVE('',#6602,#6601,#5698,.T.);
#8402=EDGE_CURVE('',#6603,#6602,#5699,.T.);
#8403=EDGE_CURVE('',#6604,#6603,#5700,.T.);
#8404=EDGE_CURVE('',#6605,#6604,#5701,.T.);
#8405=EDGE_CURVE('',#6606,#6605,#5702,.T.);
#8406=EDGE_CURVE('',#6607,#6606,#5703,.T.);
#8407=EDGE_CURVE('',#6608,#6607,#5704,.T.);
#8408=EDGE_CURVE('',#6609,#6608,#5705,.T.);
#8409=EDGE_CURVE('',#6610,#6609,#5706,.T.);
#8410=EDGE_CURVE('',#6611,#6610,#5707,.T.);
#8411=EDGE_CURVE('',#6612,#6611,#5708,.T.);
#8412=EDGE_CURVE('',#6613,#6612,#5709,.T.);
#8413=EDGE_CURVE('',#6614,#6613,#5710,.T.);
#8414=EDGE_CURVE('',#6615,#6614,#5711,.T.);
#8415=EDGE_CURVE('',#6616,#6615,#5712,.T.);
#8416=EDGE_CURVE('',#6617,#6616,#5713,.T.);
#8417=EDGE_CURVE('',#6618,#6617,#5714,.T.);
#8418=EDGE_CURVE('',#6619,#6618,#5715,.T.);
#8419=EDGE_CURVE('',#6620,#6619,#5716,.T.);
#8420=EDGE_CURVE('',#6621,#6620,#5717,.T.);
#8421=EDGE_CURVE('',#6622,#6621,#5718,.T.);
#8422=EDGE_CURVE('',#6623,#6622,#5719,.T.);
#8423=EDGE_CURVE('',#6624,#6623,#5720,.T.);
#8424=EDGE_CURVE('',#6625,#6624,#5721,.T.);
#8425=EDGE_CURVE('',#6626,#6625,#5722,.T.);
#8426=EDGE_CURVE('',#6627,#6626,#5723,.T.);
#8427=EDGE_CURVE('',#6628,#6627,#5724,.T.);
#8428=EDGE_CURVE('',#6629,#6628,#5725,.T.);
#8429=EDGE_CURVE('',#6630,#6629,#5726,.T.);
#8430=EDGE_CURVE('',#6631,#6630,#5727,.T.);
#8431=EDGE_CURVE('',#6632,#6631,#5728,.T.);
#8432=EDGE_CURVE('',#6633,#6632,#5729,.T.);
#8433=EDGE_CURVE('',#6634,#6633,#5730,.T.);
#8434=EDGE_CURVE('',#6635,#6634,#5731,.T.);
#8435=EDGE_CURVE('',#6636,#6635,#5732,.T.);
#8436=EDGE_CURVE('',#6637,#6636,#5733,.T.);
#8437=EDGE_CURVE('',#6638,#6637,#5734,.T.);
#8438=EDGE_CURVE('',#6639,#6638,#5735,.T.);
#8439=EDGE_CURVE('',#6640,#6639,#5736,.T.);
#8440=EDGE_CURVE('',#6641,#6640,#5737,.T.);
#8441=EDGE_CURVE('',#6642,#6641,#5738,.T.);
#8442=EDGE_CURVE('',#6643,#6642,#5739,.T.);
#8443=EDGE_CURVE('',#6644,#6643,#5740,.T.);
#8444=EDGE_CURVE('',#6645,#6644,#5741,.T.);
#8445=EDGE_CURVE('',#6646,#6645,#5742,.T.);
#8446=EDGE_CURVE('',#6647,#6646,#5743,.T.);
#8447=EDGE_CURVE('',#6648,#6647,#5744,.T.);
#8448=EDGE_CURVE('',#6649,#6648,#5745,.T.);
#8449=EDGE_CURVE('',#6650,#6649,#5746,.T.);
#8450=EDGE_CURVE('',#6651,#6650,#5747,.T.);
#8451=EDGE_CURVE('',#6652,#6651,#5748,.T.);
#8452=EDGE_CURVE('',#6653,#6652,#5749,.T.);
#8453=EDGE_CURVE('',#6654,#6653,#5750,.T.);
#8454=EDGE_CURVE('',#6655,#6654,#5751,.T.);
#8455=EDGE_CURVE('',#6656,#6655,#5752,.T.);
#8456=EDGE_CURVE('',#6657,#6656,#5753,.T.);
#8457=EDGE_CURVE('',#6658,#6657,#5754,.T.);
#8458=EDGE_CURVE('',#6659,#6658,#5755,.T.);
#8459=EDGE_CURVE('',#6660,#6659,#5756,.T.);
#8460=EDGE_CURVE('',#6661,#6660,#5757,.T.);
#8461=EDGE_CURVE('',#6662,#6661,#5758,.T.);
#8462=EDGE_CURVE('',#6663,#6662,#5759,.T.);
#8463=EDGE_CURVE('',#6664,#6663,#5760,.T.);
#8464=EDGE_CURVE('',#6665,#6664,#5761,.T.);
#8465=EDGE_CURVE('',#6666,#6665,#5762,.T.);
#8466=EDGE_CURVE('',#6667,#6666,#5763,.T.);
#8467=EDGE_CURVE('',#6668,#6667,#5764,.T.);
#8468=EDGE_CURVE('',#6669,#6668,#5765,.T.);
#8469=EDGE_CURVE('',#6670,#6669,#5766,.T.);
#8470=EDGE_CURVE('',#6671,#6670,#5767,.T.);
#8471=EDGE_CURVE('',#6672,#6671,#5768,.T.);
#8472=EDGE_CURVE('',#6673,#6672,#5769,.T.);
#8473=EDGE_CURVE('',#6674,#6673,#5770,.T.);
#8474=EDGE_CURVE('',#6675,#6674,#5771,.T.);
#8475=EDGE_CURVE('',#6676,#6675,#5772,.T.);
#8476=EDGE_CURVE('',#6677,#6676,#5773,.T.);
#8477=EDGE_CURVE('',#6678,#6677,#5774,.T.);
#8478=EDGE_CURVE('',#6679,#6678,#5775,.T.);
#8479=EDGE_CURVE('',#6680,#6679,#5776,.T.);
#8480=EDGE_CURVE('',#6681,#6680,#5777,.T.);
#8481=EDGE_CURVE('',#6682,#6681,#5778,.T.);
#8482=EDGE_CURVE('',#6683,#6682,#5779,.T.);
#8483=EDGE_CURVE('',#6684,#6683,#5780,.T.);
#8484=EDGE_CURVE('',#6685,#6684,#5781,.T.);
#8485=EDGE_CURVE('',#6686,#6685,#5782,.T.);
#8486=EDGE_CURVE('',#6687,#6686,#5783,.T.);
#8487=EDGE_CURVE('',#6688,#6687,#5784,.T.);
#8488=EDGE_CURVE('',#6689,#6688,#5785,.T.);
#8489=EDGE_CURVE('',#6690,#6689,#5786,.T.);
#8490=EDGE_CURVE('',#6691,#6690,#5787,.T.);
#8491=EDGE_CURVE('',#6692,#6691,#5788,.T.);
#8492=EDGE_CURVE('',#6693,#6692,#5789,.T.);
#8493=EDGE_CURVE('',#6694,#6693,#5790,.T.);
#8494=EDGE_CURVE('',#6695,#6694,#5791,.T.);
#8495=EDGE_CURVE('',#6696,#6695,#5792,.T.);
#8496=EDGE_CURVE('',#6697,#6696,#5793,.T.);
#8497=EDGE_CURVE('',#6698,#6697,#5794,.T.);
#8498=EDGE_CURVE('',#6699,#6698,#5795,.T.);
#8499=EDGE_CURVE('',#6700,#6699,#5796,.T.);
#8500=EDGE_CURVE('',#6701,#6700,#5797,.T.);
#8501=EDGE_CURVE('',#6702,#6701,#5798,.T.);
#8502=EDGE_CURVE('',#6703,#6702,#5799,.T.);
#8503=EDGE_CURVE('',#6704,#6703,#5800,.T.);
#8504=EDGE_CURVE('',#6705,#6704,#5801,.T.);
#8505=EDGE_CURVE('',#6706,#6705,#5802,.T.);
#8506=EDGE_CURVE('',#6707,#6706,#5803,.T.);
#8507=EDGE_CURVE('',#6708,#6707,#5804,.T.);
#8508=EDGE_CURVE('',#6709,#6708,#5805,.T.);
#8509=EDGE_CURVE('',#6527,#6709,#5806,.T.);
#8510=EDGE_CURVE('',#6710,#6710,#5807,.F.);
#8511=EDGE_CURVE('',#6527,#6711,#1815,.T.);
#8512=EDGE_CURVE('',#6712,#6709,#1816,.F.);
#8513=EDGE_CURVE('',#6711,#6712,#5808,.T.);
#8514=EDGE_CURVE('',#6713,#6529,#1817,.F.);
#8515=EDGE_CURVE('',#6714,#6713,#5809,.T.);
#8516=EDGE_CURVE('',#6530,#6714,#1818,.T.);
#8517=EDGE_CURVE('',#6706,#6715,#1819,.T.);
#8518=EDGE_CURVE('',#6716,#6705,#1820,.F.);
#8519=EDGE_CURVE('',#6715,#6716,#5810,.T.);
#8520=EDGE_CURVE('',#6702,#6717,#1821,.T.);
#8521=EDGE_CURVE('',#6718,#6701,#1822,.F.);
#8522=EDGE_CURVE('',#6717,#6718,#5811,.T.);
#8523=EDGE_CURVE('',#6690,#6719,#1823,.T.);
#8524=EDGE_CURVE('',#6720,#6689,#1824,.F.);
#8525=EDGE_CURVE('',#6719,#6720,#5812,.T.);
#8526=EDGE_CURVE('',#6721,#6693,#1825,.F.);
#8527=EDGE_CURVE('',#6722,#6721,#5813,.T.);
#8528=EDGE_CURVE('',#6694,#6722,#1826,.T.);
#8529=EDGE_CURVE('',#6723,#6697,#1827,.F.);
#8530=EDGE_CURVE('',#6724,#6723,#5814,.T.);
#8531=EDGE_CURVE('',#6698,#6724,#1828,.T.);
#8532=EDGE_CURVE('',#6678,#6725,#1829,.T.);
#8533=EDGE_CURVE('',#6726,#6677,#1830,.F.);
#8534=EDGE_CURVE('',#6725,#6726,#5815,.T.);
#8535=EDGE_CURVE('',#6727,#6681,#1831,.F.);
#8536=EDGE_CURVE('',#6728,#6727,#5816,.T.);
#8537=EDGE_CURVE('',#6682,#6728,#1832,.T.);
#8538=EDGE_CURVE('',#6686,#6729,#1833,.T.);
#8539=EDGE_CURVE('',#6730,#6685,#1834,.F.);
#8540=EDGE_CURVE('',#6729,#6730,#5817,.T.);
#8541=EDGE_CURVE('',#6674,#6731,#1835,.T.);
#8542=EDGE_CURVE('',#6732,#6673,#1836,.F.);
#8543=EDGE_CURVE('',#6731,#6732,#5818,.T.);
#8544=EDGE_CURVE('',#6670,#6733,#1837,.T.);
#8545=EDGE_CURVE('',#6734,#6669,#1838,.F.);
#8546=EDGE_CURVE('',#6733,#6734,#5819,.T.);
#8547=EDGE_CURVE('',#6570,#6735,#1839,.T.);
#8548=EDGE_CURVE('',#6736,#6569,#1840,.F.);
#8549=EDGE_CURVE('',#6735,#6736,#5820,.T.);
#8550=EDGE_CURVE('',#6737,#6573,#1841,.F.);
#8551=EDGE_CURVE('',#6738,#6737,#5821,.T.);
#8552=EDGE_CURVE('',#6574,#6738,#1842,.T.);
#8553=EDGE_CURVE('',#6566,#6739,#1843,.T.);
#8554=EDGE_CURVE('',#6740,#6565,#1844,.F.);
#8555=EDGE_CURVE('',#6739,#6740,#5822,.T.);
#8556=EDGE_CURVE('',#6562,#6741,#1845,.T.);
#8557=EDGE_CURVE('',#6742,#6561,#1846,.F.);
#8558=EDGE_CURVE('',#6741,#6742,#5823,.T.);
#8559=EDGE_CURVE('',#6550,#6743,#1847,.T.);
#8560=EDGE_CURVE('',#6744,#6549,#1848,.F.);
#8561=EDGE_CURVE('',#6743,#6744,#5824,.T.);
#8562=EDGE_CURVE('',#6745,#6553,#1849,.F.);
#8563=EDGE_CURVE('',#6746,#6745,#5825,.T.);
#8564=EDGE_CURVE('',#6554,#6746,#1850,.T.);
#8565=EDGE_CURVE('',#6747,#6557,#1851,.F.);
#8566=EDGE_CURVE('',#6748,#6747,#5826,.T.);
#8567=EDGE_CURVE('',#6558,#6748,#1852,.T.);
#8568=EDGE_CURVE('',#6538,#6749,#1853,.T.);
#8569=EDGE_CURVE('',#6750,#6537,#1854,.F.);
#8570=EDGE_CURVE('',#6749,#6750,#5827,.T.);
#8571=EDGE_CURVE('',#6751,#6541,#1855,.F.);
#8572=EDGE_CURVE('',#6752,#6751,#5828,.T.);
#8573=EDGE_CURVE('',#6542,#6752,#1856,.T.);
#8574=EDGE_CURVE('',#6546,#6753,#1857,.T.);
#8575=EDGE_CURVE('',#6754,#6545,#1858,.F.);
#8576=EDGE_CURVE('',#6753,#6754,#5829,.T.);
#8577=EDGE_CURVE('',#6534,#6755,#1859,.T.);
#8578=EDGE_CURVE('',#6756,#6533,#1860,.F.);
#8579=EDGE_CURVE('',#6755,#6756,#5830,.T.);
#8580=EDGE_CURVE('',#6614,#6757,#1861,.T.);
#8581=EDGE_CURVE('',#6758,#6613,#1862,.F.);
#8582=EDGE_CURVE('',#6757,#6758,#5831,.T.);
#8583=EDGE_CURVE('',#6759,#6617,#1863,.F.);
#8584=EDGE_CURVE('',#6760,#6759,#5832,.T.);
#8585=EDGE_CURVE('',#6618,#6760,#1864,.T.);
#8586=EDGE_CURVE('',#6610,#6761,#1865,.T.);
#8587=EDGE_CURVE('',#6762,#6609,#1866,.F.);
#8588=EDGE_CURVE('',#6761,#6762,#5833,.T.);
#8589=EDGE_CURVE('',#6606,#6763,#1867,.T.);
#8590=EDGE_CURVE('',#6764,#6605,#1868,.F.);
#8591=EDGE_CURVE('',#6763,#6764,#5834,.T.);
#8592=EDGE_CURVE('',#6594,#6765,#1869,.T.);
#8593=EDGE_CURVE('',#6766,#6593,#1870,.F.);
#8594=EDGE_CURVE('',#6765,#6766,#5835,.T.);
#8595=EDGE_CURVE('',#6767,#6597,#1871,.F.);
#8596=EDGE_CURVE('',#6768,#6767,#5836,.T.);
#8597=EDGE_CURVE('',#6598,#6768,#1872,.T.);
#8598=EDGE_CURVE('',#6602,#6769,#1873,.T.);
#8599=EDGE_CURVE('',#6770,#6601,#1874,.F.);
#8600=EDGE_CURVE('',#6769,#6770,#5837,.T.);
#8601=EDGE_CURVE('',#6586,#6771,#1875,.T.);
#8602=EDGE_CURVE('',#6772,#6585,#1876,.F.);
#8603=EDGE_CURVE('',#6771,#6772,#5838,.T.);
#8604=EDGE_CURVE('',#6773,#6589,#1877,.F.);
#8605=EDGE_CURVE('',#6774,#6773,#5839,.T.);
#8606=EDGE_CURVE('',#6590,#6774,#1878,.T.);
#8607=EDGE_CURVE('',#6582,#6775,#1879,.T.);
#8608=EDGE_CURVE('',#6776,#6581,#1880,.F.);
#8609=EDGE_CURVE('',#6775,#6776,#5840,.T.);
#8610=EDGE_CURVE('',#6578,#6777,#1881,.T.);
#8611=EDGE_CURVE('',#6778,#6577,#1882,.F.);
#8612=EDGE_CURVE('',#6777,#6778,#5841,.T.);
#8613=EDGE_CURVE('',#6658,#6779,#1883,.T.);
#8614=EDGE_CURVE('',#6780,#6657,#1884,.F.);
#8615=EDGE_CURVE('',#6779,#6780,#5842,.T.);
#8616=EDGE_CURVE('',#6781,#6661,#1885,.F.);
#8617=EDGE_CURVE('',#6782,#6781,#5843,.T.);
#8618=EDGE_CURVE('',#6662,#6782,#1886,.T.);
#8619=EDGE_CURVE('',#6654,#6783,#1887,.T.);
#8620=EDGE_CURVE('',#6784,#6653,#1888,.F.);
#8621=EDGE_CURVE('',#6783,#6784,#5844,.T.);
#8622=EDGE_CURVE('',#6650,#6785,#1889,.T.);
#8623=EDGE_CURVE('',#6786,#6649,#1890,.F.);
#8624=EDGE_CURVE('',#6785,#6786,#5845,.T.);
#8625=EDGE_CURVE('',#6638,#6787,#1891,.T.);
#8626=EDGE_CURVE('',#6788,#6637,#1892,.F.);
#8627=EDGE_CURVE('',#6787,#6788,#5846,.T.);
#8628=EDGE_CURVE('',#6789,#6641,#1893,.F.);
#8629=EDGE_CURVE('',#6790,#6789,#5847,.T.);
#8630=EDGE_CURVE('',#6642,#6790,#1894,.T.);
#8631=EDGE_CURVE('',#6646,#6791,#1895,.T.);
#8632=EDGE_CURVE('',#6792,#6645,#1896,.F.);
#8633=EDGE_CURVE('',#6791,#6792,#5848,.T.);
#8634=EDGE_CURVE('',#6630,#6793,#1897,.T.);
#8635=EDGE_CURVE('',#6794,#6629,#1898,.F.);
#8636=EDGE_CURVE('',#6793,#6794,#5849,.T.);
#8637=EDGE_CURVE('',#6795,#6633,#1899,.F.);
#8638=EDGE_CURVE('',#6796,#6795,#5850,.T.);
#8639=EDGE_CURVE('',#6634,#6796,#1900,.T.);
#8640=EDGE_CURVE('',#6626,#6797,#1901,.T.);
#8641=EDGE_CURVE('',#6798,#6625,#1902,.F.);
#8642=EDGE_CURVE('',#6797,#6798,#5851,.T.);
#8643=EDGE_CURVE('',#6622,#6799,#1903,.T.);
#8644=EDGE_CURVE('',#6800,#6621,#1904,.F.);
#8645=EDGE_CURVE('',#6799,#6800,#5852,.T.);
#8646=EDGE_CURVE('',#6801,#6711,#5853,.T.);
#8647=EDGE_CURVE('',#6802,#6712,#5854,.T.);
#8648=EDGE_CURVE('',#6802,#6803,#5855,.T.);
#8649=EDGE_CURVE('',#6803,#6715,#5856,.T.);
#8650=EDGE_CURVE('',#6804,#6716,#5857,.T.);
#8651=EDGE_CURVE('',#6804,#6805,#5858,.T.);
#8652=EDGE_CURVE('',#6805,#6717,#5859,.T.);
#8653=EDGE_CURVE('',#6806,#6718,#5860,.T.);
#8654=EDGE_CURVE('',#6806,#6807,#5861,.T.);
#8655=EDGE_CURVE('',#6807,#6724,#5862,.T.);
#8656=EDGE_CURVE('',#6808,#6723,#5863,.T.);
#8657=EDGE_CURVE('',#6808,#6809,#5864,.T.);
#8658=EDGE_CURVE('',#6809,#6722,#5865,.T.);
#8659=EDGE_CURVE('',#6810,#6721,#5866,.T.);
#8660=EDGE_CURVE('',#6810,#6811,#5867,.T.);
#8661=EDGE_CURVE('',#6811,#6719,#5868,.T.);
#8662=EDGE_CURVE('',#6812,#6720,#5869,.T.);
#8663=EDGE_CURVE('',#6812,#6813,#5870,.T.);
#8664=EDGE_CURVE('',#6813,#6729,#5871,.T.);
#8665=EDGE_CURVE('',#6814,#6730,#5872,.T.);
#8666=EDGE_CURVE('',#6814,#6815,#5873,.T.);
#8667=EDGE_CURVE('',#6815,#6728,#5874,.T.);
#8668=EDGE_CURVE('',#6816,#6727,#5875,.T.);
#8669=EDGE_CURVE('',#6816,#6817,#5876,.T.);
#8670=EDGE_CURVE('',#6817,#6725,#5877,.T.);
#8671=EDGE_CURVE('',#6818,#6726,#5878,.T.);
#8672=EDGE_CURVE('',#6818,#6819,#5879,.T.);
#8673=EDGE_CURVE('',#6819,#6731,#5880,.T.);
#8674=EDGE_CURVE('',#6820,#6732,#5881,.T.);
#8675=EDGE_CURVE('',#6820,#6821,#5882,.T.);
#8676=EDGE_CURVE('',#6821,#6733,#5883,.T.);
#8677=EDGE_CURVE('',#6822,#6734,#5884,.T.);
#8678=EDGE_CURVE('',#6822,#6823,#5885,.T.);
#8679=EDGE_CURVE('',#6823,#6824,#5886,.T.);
#8680=EDGE_CURVE('',#6824,#6825,#5887,.T.);
#8681=EDGE_CURVE('',#6826,#6825,#5888,.T.);
#8682=EDGE_CURVE('',#6826,#6827,#5889,.T.);
#8683=EDGE_CURVE('',#6827,#6782,#5890,.T.);
#8684=EDGE_CURVE('',#6828,#6781,#5891,.T.);
#8685=EDGE_CURVE('',#6828,#6829,#5892,.T.);
#8686=EDGE_CURVE('',#6829,#6779,#5893,.T.);
#8687=EDGE_CURVE('',#6830,#6780,#5894,.T.);
#8688=EDGE_CURVE('',#6830,#6831,#5895,.T.);
#8689=EDGE_CURVE('',#6831,#6783,#5896,.T.);
#8690=EDGE_CURVE('',#6832,#6784,#5897,.T.);
#8691=EDGE_CURVE('',#6832,#6833,#5898,.T.);
#8692=EDGE_CURVE('',#6833,#6785,#5899,.T.);
#8693=EDGE_CURVE('',#6834,#6786,#5900,.T.);
#8694=EDGE_CURVE('',#6834,#6835,#5901,.T.);
#8695=EDGE_CURVE('',#6835,#6791,#5902,.T.);
#8696=EDGE_CURVE('',#6836,#6792,#5903,.T.);
#8697=EDGE_CURVE('',#6836,#6837,#5904,.T.);
#8698=EDGE_CURVE('',#6837,#6790,#5905,.T.);
#8699=EDGE_CURVE('',#6838,#6789,#5906,.T.);
#8700=EDGE_CURVE('',#6838,#6839,#5907,.T.);
#8701=EDGE_CURVE('',#6839,#6787,#5908,.T.);
#8702=EDGE_CURVE('',#6840,#6788,#5909,.T.);
#8703=EDGE_CURVE('',#6840,#6841,#5910,.T.);
#8704=EDGE_CURVE('',#6841,#6796,#5911,.T.);
#8705=EDGE_CURVE('',#6842,#6795,#5912,.T.);
#8706=EDGE_CURVE('',#6842,#6843,#5913,.T.);
#8707=EDGE_CURVE('',#6843,#6793,#5914,.T.);
#8708=EDGE_CURVE('',#6844,#6794,#5915,.T.);
#8709=EDGE_CURVE('',#6844,#6845,#5916,.T.);
#8710=EDGE_CURVE('',#6845,#6797,#5917,.T.);
#8711=EDGE_CURVE('',#6846,#6798,#5918,.T.);
#8712=EDGE_CURVE('',#6846,#6847,#5919,.T.);
#8713=EDGE_CURVE('',#6847,#6799,#5920,.T.);
#8714=EDGE_CURVE('',#6848,#6800,#5921,.T.);
#8715=EDGE_CURVE('',#6848,#6849,#5922,.T.);
#8716=EDGE_CURVE('',#6849,#6760,#5923,.T.);
#8717=EDGE_CURVE('',#6850,#6759,#5924,.T.);
#8718=EDGE_CURVE('',#6850,#6851,#5925,.T.);
#8719=EDGE_CURVE('',#6851,#6757,#5926,.T.);
#8720=EDGE_CURVE('',#6852,#6758,#5927,.T.);
#8721=EDGE_CURVE('',#6852,#6853,#5928,.T.);
#8722=EDGE_CURVE('',#6853,#6761,#5929,.T.);
#8723=EDGE_CURVE('',#6854,#6762,#5930,.T.);
#8724=EDGE_CURVE('',#6854,#6855,#5931,.T.);
#8725=EDGE_CURVE('',#6855,#6763,#5932,.T.);
#8726=EDGE_CURVE('',#6856,#6764,#5933,.T.);
#8727=EDGE_CURVE('',#6856,#6857,#5934,.T.);
#8728=EDGE_CURVE('',#6857,#6769,#5935,.T.);
#8729=EDGE_CURVE('',#6858,#6770,#5936,.T.);
#8730=EDGE_CURVE('',#6858,#6859,#5937,.T.);
#8731=EDGE_CURVE('',#6859,#6768,#5938,.T.);
#8732=EDGE_CURVE('',#6860,#6767,#5939,.T.);
#8733=EDGE_CURVE('',#6860,#6861,#5940,.T.);
#8734=EDGE_CURVE('',#6861,#6765,#5941,.T.);
#8735=EDGE_CURVE('',#6862,#6766,#5942,.T.);
#8736=EDGE_CURVE('',#6862,#6863,#5943,.T.);
#8737=EDGE_CURVE('',#6863,#6774,#5944,.T.);
#8738=EDGE_CURVE('',#6864,#6773,#5945,.T.);
#8739=EDGE_CURVE('',#6864,#6865,#5946,.T.);
#8740=EDGE_CURVE('',#6865,#6771,#5947,.T.);
#8741=EDGE_CURVE('',#6866,#6772,#5948,.T.);
#8742=EDGE_CURVE('',#6866,#6867,#5949,.T.);
#8743=EDGE_CURVE('',#6867,#6775,#5950,.T.);
#8744=EDGE_CURVE('',#6868,#6776,#5951,.T.);
#8745=EDGE_CURVE('',#6868,#6869,#5952,.T.);
#8746=EDGE_CURVE('',#6869,#6777,#5953,.T.);
#8747=EDGE_CURVE('',#6870,#6778,#5954,.T.);
#8748=EDGE_CURVE('',#6870,#6871,#5955,.T.);
#8749=EDGE_CURVE('',#6871,#6738,#5956,.T.);
#8750=EDGE_CURVE('',#6872,#6737,#5957,.T.);
#8751=EDGE_CURVE('',#6872,#6873,#5958,.T.);
#8752=EDGE_CURVE('',#6873,#6735,#5959,.T.);
#8753=EDGE_CURVE('',#6874,#6736,#5960,.T.);
#8754=EDGE_CURVE('',#6874,#6875,#5961,.T.);
#8755=EDGE_CURVE('',#6875,#6739,#5962,.T.);
#8756=EDGE_CURVE('',#6876,#6740,#5963,.T.);
#8757=EDGE_CURVE('',#6876,#6877,#5964,.T.);
#8758=EDGE_CURVE('',#6877,#6741,#5965,.T.);
#8759=EDGE_CURVE('',#6878,#6742,#5966,.T.);
#8760=EDGE_CURVE('',#6878,#6879,#5967,.T.);
#8761=EDGE_CURVE('',#6879,#6748,#5968,.T.);
#8762=EDGE_CURVE('',#6880,#6747,#5969,.T.);
#8763=EDGE_CURVE('',#6880,#6881,#5970,.T.);
#8764=EDGE_CURVE('',#6881,#6746,#5971,.T.);
#8765=EDGE_CURVE('',#6882,#6745,#5972,.T.);
#8766=EDGE_CURVE('',#6882,#6883,#5973,.T.);
#8767=EDGE_CURVE('',#6883,#6743,#5974,.T.);
#8768=EDGE_CURVE('',#6884,#6744,#5975,.T.);
#8769=EDGE_CURVE('',#6884,#6885,#5976,.T.);
#8770=EDGE_CURVE('',#6885,#6753,#5977,.T.);
#8771=EDGE_CURVE('',#6886,#6754,#5978,.T.);
#8772=EDGE_CURVE('',#6886,#6887,#5979,.T.);
#8773=EDGE_CURVE('',#6887,#6752,#5980,.T.);
#8774=EDGE_CURVE('',#6888,#6751,#5981,.T.);
#8775=EDGE_CURVE('',#6888,#6889,#5982,.T.);
#8776=EDGE_CURVE('',#6889,#6749,#5983,.T.);
#8777=EDGE_CURVE('',#6890,#6750,#5984,.T.);
#8778=EDGE_CURVE('',#6890,#6891,#5985,.T.);
#8779=EDGE_CURVE('',#6891,#6755,#5986,.T.);
#8780=EDGE_CURVE('',#6892,#6756,#5987,.T.);
#8781=EDGE_CURVE('',#6892,#6893,#5988,.T.);
#8782=EDGE_CURVE('',#6893,#6714,#5989,.T.);
#8783=EDGE_CURVE('',#6894,#6713,#5990,.T.);
#8784=EDGE_CURVE('',#6894,#6801,#5991,.T.);
#8785=EDGE_CURVE('',#6895,#6895,#5992,.F.);
#8786=EDGE_CURVE('',#6666,#6824,#1905,.T.);
#8787=EDGE_CURVE('',#6825,#6665,#1906,.F.);
#8788=EDGE_CURVE('',#6663,#6827,#1907,.T.);
#8789=EDGE_CURVE('',#6664,#6826,#1908,.T.);
#8790=EDGE_CURVE('',#6667,#6823,#1909,.T.);
#8791=EDGE_CURVE('',#6668,#6822,#1910,.T.);
#8792=EDGE_CURVE('',#6619,#6849,#1911,.T.);
#8793=EDGE_CURVE('',#6620,#6848,#1912,.T.);
#8794=EDGE_CURVE('',#6623,#6847,#1913,.T.);
#8795=EDGE_CURVE('',#6624,#6846,#1914,.T.);
#8796=EDGE_CURVE('',#6627,#6845,#1915,.T.);
#8797=EDGE_CURVE('',#6628,#6844,#1916,.T.);
#8798=EDGE_CURVE('',#6635,#6841,#1917,.T.);
#8799=EDGE_CURVE('',#6636,#6840,#1918,.T.);
#8800=EDGE_CURVE('',#6631,#6843,#1919,.T.);
#8801=EDGE_CURVE('',#6632,#6842,#1920,.T.);
#8802=EDGE_CURVE('',#6643,#6837,#1921,.T.);
#8803=EDGE_CURVE('',#6644,#6836,#1922,.T.);
#8804=EDGE_CURVE('',#6647,#6835,#1923,.T.);
#8805=EDGE_CURVE('',#6648,#6834,#1924,.T.);
#8806=EDGE_CURVE('',#6639,#6839,#1925,.T.);
#8807=EDGE_CURVE('',#6640,#6838,#1926,.T.);
#8808=EDGE_CURVE('',#6651,#6833,#1927,.T.);
#8809=EDGE_CURVE('',#6652,#6832,#1928,.T.);
#8810=EDGE_CURVE('',#6655,#6831,#1929,.T.);
#8811=EDGE_CURVE('',#6656,#6830,#1930,.T.);
#8812=EDGE_CURVE('',#6659,#6829,#1931,.T.);
#8813=EDGE_CURVE('',#6660,#6828,#1932,.T.);
#8814=EDGE_CURVE('',#6575,#6871,#1933,.T.);
#8815=EDGE_CURVE('',#6576,#6870,#1934,.T.);
#8816=EDGE_CURVE('',#6579,#6869,#1935,.T.);
#8817=EDGE_CURVE('',#6580,#6868,#1936,.T.);
#8818=EDGE_CURVE('',#6583,#6867,#1937,.T.);
#8819=EDGE_CURVE('',#6584,#6866,#1938,.T.);
#8820=EDGE_CURVE('',#6591,#6863,#1939,.T.);
#8821=EDGE_CURVE('',#6592,#6862,#1940,.T.);
#8822=EDGE_CURVE('',#6587,#6865,#1941,.T.);
#8823=EDGE_CURVE('',#6588,#6864,#1942,.T.);
#8824=EDGE_CURVE('',#6599,#6859,#1943,.T.);
#8825=EDGE_CURVE('',#6600,#6858,#1944,.T.);
#8826=EDGE_CURVE('',#6603,#6857,#1945,.T.);
#8827=EDGE_CURVE('',#6604,#6856,#1946,.T.);
#8828=EDGE_CURVE('',#6595,#6861,#1947,.T.);
#8829=EDGE_CURVE('',#6596,#6860,#1948,.T.);
#8830=EDGE_CURVE('',#6607,#6855,#1949,.T.);
#8831=EDGE_CURVE('',#6608,#6854,#1950,.T.);
#8832=EDGE_CURVE('',#6611,#6853,#1951,.T.);
#8833=EDGE_CURVE('',#6612,#6852,#1952,.T.);
#8834=EDGE_CURVE('',#6615,#6851,#1953,.T.);
#8835=EDGE_CURVE('',#6616,#6850,#1954,.T.);
#8836=EDGE_CURVE('',#6531,#6893,#1955,.T.);
#8837=EDGE_CURVE('',#6532,#6892,#1956,.T.);
#8838=EDGE_CURVE('',#6535,#6891,#1957,.T.);
#8839=EDGE_CURVE('',#6536,#6890,#1958,.T.);
#8840=EDGE_CURVE('',#6543,#6887,#1959,.T.);
#8841=EDGE_CURVE('',#6544,#6886,#1960,.T.);
#8842=EDGE_CURVE('',#6547,#6885,#1961,.T.);
#8843=EDGE_CURVE('',#6548,#6884,#1962,.T.);
#8844=EDGE_CURVE('',#6539,#6889,#1963,.T.);
#8845=EDGE_CURVE('',#6540,#6888,#1964,.T.);
#8846=EDGE_CURVE('',#6559,#6879,#1965,.T.);
#8847=EDGE_CURVE('',#6560,#6878,#1966,.T.);
#8848=EDGE_CURVE('',#6555,#6881,#1967,.T.);
#8849=EDGE_CURVE('',#6556,#6880,#1968,.T.);
#8850=EDGE_CURVE('',#6551,#6883,#1969,.T.);
#8851=EDGE_CURVE('',#6552,#6882,#1970,.T.);
#8852=EDGE_CURVE('',#6563,#6877,#1971,.T.);
#8853=EDGE_CURVE('',#6564,#6876,#1972,.T.);
#8854=EDGE_CURVE('',#6567,#6875,#1973,.T.);
#8855=EDGE_CURVE('',#6568,#6874,#1974,.T.);
#8856=EDGE_CURVE('',#6571,#6873,#1975,.T.);
#8857=EDGE_CURVE('',#6572,#6872,#1976,.T.);
#8858=EDGE_CURVE('',#6671,#6821,#1977,.T.);
#8859=EDGE_CURVE('',#6672,#6820,#1978,.T.);
#8860=EDGE_CURVE('',#6675,#6819,#1979,.T.);
#8861=EDGE_CURVE('',#6676,#6818,#1980,.T.);
#8862=EDGE_CURVE('',#6683,#6815,#1981,.T.);
#8863=EDGE_CURVE('',#6684,#6814,#1982,.T.);
#8864=EDGE_CURVE('',#6687,#6813,#1983,.T.);
#8865=EDGE_CURVE('',#6688,#6812,#1984,.T.);
#8866=EDGE_CURVE('',#6679,#6817,#1985,.T.);
#8867=EDGE_CURVE('',#6680,#6816,#1986,.T.);
#8868=EDGE_CURVE('',#6699,#6807,#1987,.T.);
#8869=EDGE_CURVE('',#6700,#6806,#1988,.T.);
#8870=EDGE_CURVE('',#6695,#6809,#1989,.T.);
#8871=EDGE_CURVE('',#6696,#6808,#1990,.T.);
#8872=EDGE_CURVE('',#6691,#6811,#1991,.T.);
#8873=EDGE_CURVE('',#6692,#6810,#1992,.T.);
#8874=EDGE_CURVE('',#6703,#6805,#1993,.T.);
#8875=EDGE_CURVE('',#6704,#6804,#1994,.T.);
#8876=EDGE_CURVE('',#6707,#6803,#1995,.T.);
#8877=EDGE_CURVE('',#6708,#6802,#1996,.T.);
#8878=EDGE_CURVE('',#6526,#6801,#1997,.T.);
#8879=EDGE_CURVE('',#6528,#6894,#1998,.T.);
#8880=EDGE_CURVE('',#6710,#6895,#1999,.T.);
#11069=ORIENTED_EDGE('',*,*,#8326,.F.);
#11070=ORIENTED_EDGE('',*,*,#8327,.F.);
#11071=ORIENTED_EDGE('',*,*,#8328,.F.);
#11072=ORIENTED_EDGE('',*,*,#8329,.F.);
#11073=ORIENTED_EDGE('',*,*,#8330,.F.);
#11074=ORIENTED_EDGE('',*,*,#8331,.F.);
#11075=ORIENTED_EDGE('',*,*,#8332,.F.);
#11076=ORIENTED_EDGE('',*,*,#8333,.F.);
#11077=ORIENTED_EDGE('',*,*,#8334,.F.);
#11078=ORIENTED_EDGE('',*,*,#8335,.F.);
#11079=ORIENTED_EDGE('',*,*,#8336,.F.);
#11080=ORIENTED_EDGE('',*,*,#8337,.F.);
#11081=ORIENTED_EDGE('',*,*,#8338,.F.);
#11082=ORIENTED_EDGE('',*,*,#8339,.F.);
#11083=ORIENTED_EDGE('',*,*,#8340,.F.);
#11084=ORIENTED_EDGE('',*,*,#8341,.F.);
#11085=ORIENTED_EDGE('',*,*,#8342,.F.);
#11086=ORIENTED_EDGE('',*,*,#8343,.F.);
#11087=ORIENTED_EDGE('',*,*,#8344,.F.);
#11088=ORIENTED_EDGE('',*,*,#8345,.F.);
#11089=ORIENTED_EDGE('',*,*,#8346,.F.);
#11090=ORIENTED_EDGE('',*,*,#8347,.F.);
#11091=ORIENTED_EDGE('',*,*,#8348,.F.);
#11092=ORIENTED_EDGE('',*,*,#8349,.F.);
#11093=ORIENTED_EDGE('',*,*,#8350,.F.);
#11094=ORIENTED_EDGE('',*,*,#8351,.F.);
#11095=ORIENTED_EDGE('',*,*,#8352,.F.);
#11096=ORIENTED_EDGE('',*,*,#8353,.F.);
#11097=ORIENTED_EDGE('',*,*,#8354,.F.);
#11098=ORIENTED_EDGE('',*,*,#8355,.F.);
#11099=ORIENTED_EDGE('',*,*,#8356,.F.);
#11100=ORIENTED_EDGE('',*,*,#8357,.F.);
#11101=ORIENTED_EDGE('',*,*,#8358,.F.);
#11102=ORIENTED_EDGE('',*,*,#8359,.F.);
#11103=ORIENTED_EDGE('',*,*,#8360,.F.);
#11104=ORIENTED_EDGE('',*,*,#8361,.F.);
#11105=ORIENTED_EDGE('',*,*,#8362,.F.);
#11106=ORIENTED_EDGE('',*,*,#8363,.F.);
#11107=ORIENTED_EDGE('',*,*,#8364,.F.);
#11108=ORIENTED_EDGE('',*,*,#8365,.F.);
#11109=ORIENTED_EDGE('',*,*,#8366,.F.);
#11110=ORIENTED_EDGE('',*,*,#8367,.F.);
#11111=ORIENTED_EDGE('',*,*,#8368,.F.);
#11112=ORIENTED_EDGE('',*,*,#8369,.F.);
#11113=ORIENTED_EDGE('',*,*,#8370,.F.);
#11114=ORIENTED_EDGE('',*,*,#8371,.F.);
#11115=ORIENTED_EDGE('',*,*,#8372,.F.);
#11116=ORIENTED_EDGE('',*,*,#8373,.F.);
#11117=ORIENTED_EDGE('',*,*,#8374,.F.);
#11118=ORIENTED_EDGE('',*,*,#8375,.F.);
#11119=ORIENTED_EDGE('',*,*,#8376,.F.);
#11120=ORIENTED_EDGE('',*,*,#8377,.F.);
#11121=ORIENTED_EDGE('',*,*,#8378,.F.);
#11122=ORIENTED_EDGE('',*,*,#8379,.F.);
#11123=ORIENTED_EDGE('',*,*,#8380,.F.);
#11124=ORIENTED_EDGE('',*,*,#8381,.F.);
#11125=ORIENTED_EDGE('',*,*,#8382,.F.);
#11126=ORIENTED_EDGE('',*,*,#8383,.F.);
#11127=ORIENTED_EDGE('',*,*,#8384,.F.);
#11128=ORIENTED_EDGE('',*,*,#8385,.F.);
#11129=ORIENTED_EDGE('',*,*,#8386,.F.);
#11130=ORIENTED_EDGE('',*,*,#8387,.F.);
#11131=ORIENTED_EDGE('',*,*,#8388,.F.);
#11132=ORIENTED_EDGE('',*,*,#8389,.F.);
#11133=ORIENTED_EDGE('',*,*,#8390,.F.);
#11134=ORIENTED_EDGE('',*,*,#8391,.F.);
#11135=ORIENTED_EDGE('',*,*,#8392,.F.);
#11136=ORIENTED_EDGE('',*,*,#8393,.F.);
#11137=ORIENTED_EDGE('',*,*,#8394,.F.);
#11138=ORIENTED_EDGE('',*,*,#8395,.F.);
#11139=ORIENTED_EDGE('',*,*,#8396,.F.);
#11140=ORIENTED_EDGE('',*,*,#8397,.F.);
#11141=ORIENTED_EDGE('',*,*,#8398,.F.);
#11142=ORIENTED_EDGE('',*,*,#8399,.F.);
#11143=ORIENTED_EDGE('',*,*,#8400,.F.);
#11144=ORIENTED_EDGE('',*,*,#8401,.F.);
#11145=ORIENTED_EDGE('',*,*,#8402,.F.);
#11146=ORIENTED_EDGE('',*,*,#8403,.F.);
#11147=ORIENTED_EDGE('',*,*,#8404,.F.);
#11148=ORIENTED_EDGE('',*,*,#8405,.F.);
#11149=ORIENTED_EDGE('',*,*,#8406,.F.);
#11150=ORIENTED_EDGE('',*,*,#8407,.F.);
#11151=ORIENTED_EDGE('',*,*,#8408,.F.);
#11152=ORIENTED_EDGE('',*,*,#8409,.F.);
#11153=ORIENTED_EDGE('',*,*,#8410,.F.);
#11154=ORIENTED_EDGE('',*,*,#8411,.F.);
#11155=ORIENTED_EDGE('',*,*,#8412,.F.);
#11156=ORIENTED_EDGE('',*,*,#8413,.F.);
#11157=ORIENTED_EDGE('',*,*,#8414,.F.);
#11158=ORIENTED_EDGE('',*,*,#8415,.F.);
#11159=ORIENTED_EDGE('',*,*,#8416,.F.);
#11160=ORIENTED_EDGE('',*,*,#8417,.F.);
#11161=ORIENTED_EDGE('',*,*,#8418,.F.);
#11162=ORIENTED_EDGE('',*,*,#8419,.F.);
#11163=ORIENTED_EDGE('',*,*,#8420,.F.);
#11164=ORIENTED_EDGE('',*,*,#8421,.F.);
#11165=ORIENTED_EDGE('',*,*,#8422,.F.);
#11166=ORIENTED_EDGE('',*,*,#8423,.F.);
#11167=ORIENTED_EDGE('',*,*,#8424,.F.);
#11168=ORIENTED_EDGE('',*,*,#8425,.F.);
#11169=ORIENTED_EDGE('',*,*,#8426,.F.);
#11170=ORIENTED_EDGE('',*,*,#8427,.F.);
#11171=ORIENTED_EDGE('',*,*,#8428,.F.);
#11172=ORIENTED_EDGE('',*,*,#8429,.F.);
#11173=ORIENTED_EDGE('',*,*,#8430,.F.);
#11174=ORIENTED_EDGE('',*,*,#8431,.F.);
#11175=ORIENTED_EDGE('',*,*,#8432,.F.);
#11176=ORIENTED_EDGE('',*,*,#8433,.F.);
#11177=ORIENTED_EDGE('',*,*,#8434,.F.);
#11178=ORIENTED_EDGE('',*,*,#8435,.F.);
#11179=ORIENTED_EDGE('',*,*,#8436,.F.);
#11180=ORIENTED_EDGE('',*,*,#8437,.F.);
#11181=ORIENTED_EDGE('',*,*,#8438,.F.);
#11182=ORIENTED_EDGE('',*,*,#8439,.F.);
#11183=ORIENTED_EDGE('',*,*,#8440,.F.);
#11184=ORIENTED_EDGE('',*,*,#8441,.F.);
#11185=ORIENTED_EDGE('',*,*,#8442,.F.);
#11186=ORIENTED_EDGE('',*,*,#8443,.F.);
#11187=ORIENTED_EDGE('',*,*,#8444,.F.);
#11188=ORIENTED_EDGE('',*,*,#8445,.F.);
#11189=ORIENTED_EDGE('',*,*,#8446,.F.);
#11190=ORIENTED_EDGE('',*,*,#8447,.F.);
#11191=ORIENTED_EDGE('',*,*,#8448,.F.);
#11192=ORIENTED_EDGE('',*,*,#8449,.F.);
#11193=ORIENTED_EDGE('',*,*,#8450,.F.);
#11194=ORIENTED_EDGE('',*,*,#8451,.F.);
#11195=ORIENTED_EDGE('',*,*,#8452,.F.);
#11196=ORIENTED_EDGE('',*,*,#8453,.F.);
#11197=ORIENTED_EDGE('',*,*,#8454,.F.);
#11198=ORIENTED_EDGE('',*,*,#8455,.F.);
#11199=ORIENTED_EDGE('',*,*,#8456,.F.);
#11200=ORIENTED_EDGE('',*,*,#8457,.F.);
#11201=ORIENTED_EDGE('',*,*,#8458,.F.);
#11202=ORIENTED_EDGE('',*,*,#8459,.F.);
#11203=ORIENTED_EDGE('',*,*,#8460,.F.);
#11204=ORIENTED_EDGE('',*,*,#8461,.F.);
#11205=ORIENTED_EDGE('',*,*,#8462,.F.);
#11206=ORIENTED_EDGE('',*,*,#8463,.F.);
#11207=ORIENTED_EDGE('',*,*,#8464,.F.);
#11208=ORIENTED_EDGE('',*,*,#8465,.F.);
#11209=ORIENTED_EDGE('',*,*,#8466,.F.);
#11210=ORIENTED_EDGE('',*,*,#8467,.F.);
#11211=ORIENTED_EDGE('',*,*,#8468,.F.);
#11212=ORIENTED_EDGE('',*,*,#8469,.F.);
#11213=ORIENTED_EDGE('',*,*,#8470,.F.);
#11214=ORIENTED_EDGE('',*,*,#8471,.F.);
#11215=ORIENTED_EDGE('',*,*,#8472,.F.);
#11216=ORIENTED_EDGE('',*,*,#8473,.F.);
#11217=ORIENTED_EDGE('',*,*,#8474,.F.);
#11218=ORIENTED_EDGE('',*,*,#8475,.F.);
#11219=ORIENTED_EDGE('',*,*,#8476,.F.);
#11220=ORIENTED_EDGE('',*,*,#8477,.F.);
#11221=ORIENTED_EDGE('',*,*,#8478,.F.);
#11222=ORIENTED_EDGE('',*,*,#8479,.F.);
#11223=ORIENTED_EDGE('',*,*,#8480,.F.);
#11224=ORIENTED_EDGE('',*,*,#8481,.F.);
#11225=ORIENTED_EDGE('',*,*,#8482,.F.);
#11226=ORIENTED_EDGE('',*,*,#8483,.F.);
#11227=ORIENTED_EDGE('',*,*,#8484,.F.);
#11228=ORIENTED_EDGE('',*,*,#8485,.F.);
#11229=ORIENTED_EDGE('',*,*,#8486,.F.);
#11230=ORIENTED_EDGE('',*,*,#8487,.F.);
#11231=ORIENTED_EDGE('',*,*,#8488,.F.);
#11232=ORIENTED_EDGE('',*,*,#8489,.F.);
#11233=ORIENTED_EDGE('',*,*,#8490,.F.);
#11234=ORIENTED_EDGE('',*,*,#8491,.F.);
#11235=ORIENTED_EDGE('',*,*,#8492,.F.);
#11236=ORIENTED_EDGE('',*,*,#8493,.F.);
#11237=ORIENTED_EDGE('',*,*,#8494,.F.);
#11238=ORIENTED_EDGE('',*,*,#8495,.F.);
#11239=ORIENTED_EDGE('',*,*,#8496,.F.);
#11240=ORIENTED_EDGE('',*,*,#8497,.F.);
#11241=ORIENTED_EDGE('',*,*,#8498,.F.);
#11242=ORIENTED_EDGE('',*,*,#8499,.F.);
#11243=ORIENTED_EDGE('',*,*,#8500,.F.);
#11244=ORIENTED_EDGE('',*,*,#8501,.F.);
#11245=ORIENTED_EDGE('',*,*,#8502,.F.);
#11246=ORIENTED_EDGE('',*,*,#8503,.F.);
#11247=ORIENTED_EDGE('',*,*,#8504,.F.);
#11248=ORIENTED_EDGE('',*,*,#8505,.F.);
#11249=ORIENTED_EDGE('',*,*,#8506,.F.);
#11250=ORIENTED_EDGE('',*,*,#8507,.F.);
#11251=ORIENTED_EDGE('',*,*,#8508,.F.);
#11252=ORIENTED_EDGE('',*,*,#8509,.F.);
#11253=ORIENTED_EDGE('',*,*,#8510,.F.);
#11254=ORIENTED_EDGE('',*,*,#8511,.F.);
#11255=ORIENTED_EDGE('',*,*,#8509,.T.);
#11256=ORIENTED_EDGE('',*,*,#8512,.F.);
#11257=ORIENTED_EDGE('',*,*,#8513,.F.);
#11258=ORIENTED_EDGE('',*,*,#8514,.F.);
#11259=ORIENTED_EDGE('',*,*,#8515,.F.);
#11260=ORIENTED_EDGE('',*,*,#8516,.F.);
#11261=ORIENTED_EDGE('',*,*,#8329,.T.);
#11262=ORIENTED_EDGE('',*,*,#8517,.F.);
#11263=ORIENTED_EDGE('',*,*,#8505,.T.);
#11264=ORIENTED_EDGE('',*,*,#8518,.F.);
#11265=ORIENTED_EDGE('',*,*,#8519,.F.);
#11266=ORIENTED_EDGE('',*,*,#8520,.F.);
#11267=ORIENTED_EDGE('',*,*,#8501,.T.);
#11268=ORIENTED_EDGE('',*,*,#8521,.F.);
#11269=ORIENTED_EDGE('',*,*,#8522,.F.);
#11270=ORIENTED_EDGE('',*,*,#8523,.F.);
#11271=ORIENTED_EDGE('',*,*,#8489,.T.);
#11272=ORIENTED_EDGE('',*,*,#8524,.F.);
#11273=ORIENTED_EDGE('',*,*,#8525,.F.);
#11274=ORIENTED_EDGE('',*,*,#8526,.F.);
#11275=ORIENTED_EDGE('',*,*,#8527,.F.);
#11276=ORIENTED_EDGE('',*,*,#8528,.F.);
#11277=ORIENTED_EDGE('',*,*,#8493,.T.);
#11278=ORIENTED_EDGE('',*,*,#8529,.F.);
#11279=ORIENTED_EDGE('',*,*,#8530,.F.);
#11280=ORIENTED_EDGE('',*,*,#8531,.F.);
#11281=ORIENTED_EDGE('',*,*,#8497,.T.);
#11282=ORIENTED_EDGE('',*,*,#8532,.F.);
#11283=ORIENTED_EDGE('',*,*,#8477,.T.);
#11284=ORIENTED_EDGE('',*,*,#8533,.F.);
#11285=ORIENTED_EDGE('',*,*,#8534,.F.);
#11286=ORIENTED_EDGE('',*,*,#8535,.F.);
#11287=ORIENTED_EDGE('',*,*,#8536,.F.);
#11288=ORIENTED_EDGE('',*,*,#8537,.F.);
#11289=ORIENTED_EDGE('',*,*,#8481,.T.);
#11290=ORIENTED_EDGE('',*,*,#8538,.F.);
#11291=ORIENTED_EDGE('',*,*,#8485,.T.);
#11292=ORIENTED_EDGE('',*,*,#8539,.F.);
#11293=ORIENTED_EDGE('',*,*,#8540,.F.);
#11294=ORIENTED_EDGE('',*,*,#8541,.F.);
#11295=ORIENTED_EDGE('',*,*,#8473,.T.);
#11296=ORIENTED_EDGE('',*,*,#8542,.F.);
#11297=ORIENTED_EDGE('',*,*,#8543,.F.);
#11298=ORIENTED_EDGE('',*,*,#8544,.F.);
#11299=ORIENTED_EDGE('',*,*,#8469,.T.);
#11300=ORIENTED_EDGE('',*,*,#8545,.F.);
#11301=ORIENTED_EDGE('',*,*,#8546,.F.);
#11302=ORIENTED_EDGE('',*,*,#8547,.F.);
#11303=ORIENTED_EDGE('',*,*,#8369,.T.);
#11304=ORIENTED_EDGE('',*,*,#8548,.F.);
#11305=ORIENTED_EDGE('',*,*,#8549,.F.);
#11306=ORIENTED_EDGE('',*,*,#8550,.F.);
#11307=ORIENTED_EDGE('',*,*,#8551,.F.);
#11308=ORIENTED_EDGE('',*,*,#8552,.F.);
#11309=ORIENTED_EDGE('',*,*,#8373,.T.);
#11310=ORIENTED_EDGE('',*,*,#8553,.F.);
#11311=ORIENTED_EDGE('',*,*,#8365,.T.);
#11312=ORIENTED_EDGE('',*,*,#8554,.F.);
#11313=ORIENTED_EDGE('',*,*,#8555,.F.);
#11314=ORIENTED_EDGE('',*,*,#8556,.F.);
#11315=ORIENTED_EDGE('',*,*,#8361,.T.);
#11316=ORIENTED_EDGE('',*,*,#8557,.F.);
#11317=ORIENTED_EDGE('',*,*,#8558,.F.);
#11318=ORIENTED_EDGE('',*,*,#8559,.F.);
#11319=ORIENTED_EDGE('',*,*,#8349,.T.);
#11320=ORIENTED_EDGE('',*,*,#8560,.F.);
#11321=ORIENTED_EDGE('',*,*,#8561,.F.);
#11322=ORIENTED_EDGE('',*,*,#8562,.F.);
#11323=ORIENTED_EDGE('',*,*,#8563,.F.);
#11324=ORIENTED_EDGE('',*,*,#8564,.F.);
#11325=ORIENTED_EDGE('',*,*,#8353,.T.);
#11326=ORIENTED_EDGE('',*,*,#8565,.F.);
#11327=ORIENTED_EDGE('',*,*,#8566,.F.);
#11328=ORIENTED_EDGE('',*,*,#8567,.F.);
#11329=ORIENTED_EDGE('',*,*,#8357,.T.);
#11330=ORIENTED_EDGE('',*,*,#8568,.F.);
#11331=ORIENTED_EDGE('',*,*,#8337,.T.);
#11332=ORIENTED_EDGE('',*,*,#8569,.F.);
#11333=ORIENTED_EDGE('',*,*,#8570,.F.);
#11334=ORIENTED_EDGE('',*,*,#8571,.F.);
#11335=ORIENTED_EDGE('',*,*,#8572,.F.);
#11336=ORIENTED_EDGE('',*,*,#8573,.F.);
#11337=ORIENTED_EDGE('',*,*,#8341,.T.);
#11338=ORIENTED_EDGE('',*,*,#8574,.F.);
#11339=ORIENTED_EDGE('',*,*,#8345,.T.);
#11340=ORIENTED_EDGE('',*,*,#8575,.F.);
#11341=ORIENTED_EDGE('',*,*,#8576,.F.);
#11342=ORIENTED_EDGE('',*,*,#8577,.F.);
#11343=ORIENTED_EDGE('',*,*,#8333,.T.);
#11344=ORIENTED_EDGE('',*,*,#8578,.F.);
#11345=ORIENTED_EDGE('',*,*,#8579,.F.);
#11346=ORIENTED_EDGE('',*,*,#8580,.F.);
#11347=ORIENTED_EDGE('',*,*,#8413,.T.);
#11348=ORIENTED_EDGE('',*,*,#8581,.F.);
#11349=ORIENTED_EDGE('',*,*,#8582,.F.);
#11350=ORIENTED_EDGE('',*,*,#8583,.F.);
#11351=ORIENTED_EDGE('',*,*,#8584,.F.);
#11352=ORIENTED_EDGE('',*,*,#8585,.F.);
#11353=ORIENTED_EDGE('',*,*,#8417,.T.);
#11354=ORIENTED_EDGE('',*,*,#8586,.F.);
#11355=ORIENTED_EDGE('',*,*,#8409,.T.);
#11356=ORIENTED_EDGE('',*,*,#8587,.F.);
#11357=ORIENTED_EDGE('',*,*,#8588,.F.);
#11358=ORIENTED_EDGE('',*,*,#8589,.F.);
#11359=ORIENTED_EDGE('',*,*,#8405,.T.);
#11360=ORIENTED_EDGE('',*,*,#8590,.F.);
#11361=ORIENTED_EDGE('',*,*,#8591,.F.);
#11362=ORIENTED_EDGE('',*,*,#8592,.F.);
#11363=ORIENTED_EDGE('',*,*,#8393,.T.);
#11364=ORIENTED_EDGE('',*,*,#8593,.F.);
#11365=ORIENTED_EDGE('',*,*,#8594,.F.);
#11366=ORIENTED_EDGE('',*,*,#8595,.F.);
#11367=ORIENTED_EDGE('',*,*,#8596,.F.);
#11368=ORIENTED_EDGE('',*,*,#8597,.F.);
#11369=ORIENTED_EDGE('',*,*,#8397,.T.);
#11370=ORIENTED_EDGE('',*,*,#8598,.F.);
#11371=ORIENTED_EDGE('',*,*,#8401,.T.);
#11372=ORIENTED_EDGE('',*,*,#8599,.F.);
#11373=ORIENTED_EDGE('',*,*,#8600,.F.);
#11374=ORIENTED_EDGE('',*,*,#8601,.F.);
#11375=ORIENTED_EDGE('',*,*,#8385,.T.);
#11376=ORIENTED_EDGE('',*,*,#8602,.F.);
#11377=ORIENTED_EDGE('',*,*,#8603,.F.);
#11378=ORIENTED_EDGE('',*,*,#8604,.F.);
#11379=ORIENTED_EDGE('',*,*,#8605,.F.);
#11380=ORIENTED_EDGE('',*,*,#8606,.F.);
#11381=ORIENTED_EDGE('',*,*,#8389,.T.);
#11382=ORIENTED_EDGE('',*,*,#8607,.F.);
#11383=ORIENTED_EDGE('',*,*,#8381,.T.);
#11384=ORIENTED_EDGE('',*,*,#8608,.F.);
#11385=ORIENTED_EDGE('',*,*,#8609,.F.);
#11386=ORIENTED_EDGE('',*,*,#8610,.F.);
#11387=ORIENTED_EDGE('',*,*,#8377,.T.);
#11388=ORIENTED_EDGE('',*,*,#8611,.F.);
#11389=ORIENTED_EDGE('',*,*,#8612,.F.);
#11390=ORIENTED_EDGE('',*,*,#8613,.F.);
#11391=ORIENTED_EDGE('',*,*,#8457,.T.);
#11392=ORIENTED_EDGE('',*,*,#8614,.F.);
#11393=ORIENTED_EDGE('',*,*,#8615,.F.);
#11394=ORIENTED_EDGE('',*,*,#8616,.F.);
#11395=ORIENTED_EDGE('',*,*,#8617,.F.);
#11396=ORIENTED_EDGE('',*,*,#8618,.F.);
#11397=ORIENTED_EDGE('',*,*,#8461,.T.);
#11398=ORIENTED_EDGE('',*,*,#8619,.F.);
#11399=ORIENTED_EDGE('',*,*,#8453,.T.);
#11400=ORIENTED_EDGE('',*,*,#8620,.F.);
#11401=ORIENTED_EDGE('',*,*,#8621,.F.);
#11402=ORIENTED_EDGE('',*,*,#8622,.F.);
#11403=ORIENTED_EDGE('',*,*,#8449,.T.);
#11404=ORIENTED_EDGE('',*,*,#8623,.F.);
#11405=ORIENTED_EDGE('',*,*,#8624,.F.);
#11406=ORIENTED_EDGE('',*,*,#8625,.F.);
#11407=ORIENTED_EDGE('',*,*,#8437,.T.);
#11408=ORIENTED_EDGE('',*,*,#8626,.F.);
#11409=ORIENTED_EDGE('',*,*,#8627,.F.);
#11410=ORIENTED_EDGE('',*,*,#8628,.F.);
#11411=ORIENTED_EDGE('',*,*,#8629,.F.);
#11412=ORIENTED_EDGE('',*,*,#8630,.F.);
#11413=ORIENTED_EDGE('',*,*,#8441,.T.);
#11414=ORIENTED_EDGE('',*,*,#8631,.F.);
#11415=ORIENTED_EDGE('',*,*,#8445,.T.);
#11416=ORIENTED_EDGE('',*,*,#8632,.F.);
#11417=ORIENTED_EDGE('',*,*,#8633,.F.);
#11418=ORIENTED_EDGE('',*,*,#8634,.F.);
#11419=ORIENTED_EDGE('',*,*,#8429,.T.);
#11420=ORIENTED_EDGE('',*,*,#8635,.F.);
#11421=ORIENTED_EDGE('',*,*,#8636,.F.);
#11422=ORIENTED_EDGE('',*,*,#8637,.F.);
#11423=ORIENTED_EDGE('',*,*,#8638,.F.);
#11424=ORIENTED_EDGE('',*,*,#8639,.F.);
#11425=ORIENTED_EDGE('',*,*,#8433,.T.);
#11426=ORIENTED_EDGE('',*,*,#8640,.F.);
#11427=ORIENTED_EDGE('',*,*,#8425,.T.);
#11428=ORIENTED_EDGE('',*,*,#8641,.F.);
#11429=ORIENTED_EDGE('',*,*,#8642,.F.);
#11430=ORIENTED_EDGE('',*,*,#8643,.F.);
#11431=ORIENTED_EDGE('',*,*,#8421,.T.);
#11432=ORIENTED_EDGE('',*,*,#8644,.F.);
#11433=ORIENTED_EDGE('',*,*,#8645,.F.);
#11434=ORIENTED_EDGE('',*,*,#8646,.T.);
#11435=ORIENTED_EDGE('',*,*,#8513,.T.);
#11436=ORIENTED_EDGE('',*,*,#8647,.F.);
#11437=ORIENTED_EDGE('',*,*,#8648,.T.);
#11438=ORIENTED_EDGE('',*,*,#8649,.T.);
#11439=ORIENTED_EDGE('',*,*,#8519,.T.);
#11440=ORIENTED_EDGE('',*,*,#8650,.F.);
#11441=ORIENTED_EDGE('',*,*,#8651,.T.);
#11442=ORIENTED_EDGE('',*,*,#8652,.T.);
#11443=ORIENTED_EDGE('',*,*,#8522,.T.);
#11444=ORIENTED_EDGE('',*,*,#8653,.F.);
#11445=ORIENTED_EDGE('',*,*,#8654,.T.);
#11446=ORIENTED_EDGE('',*,*,#8655,.T.);
#11447=ORIENTED_EDGE('',*,*,#8530,.T.);
#11448=ORIENTED_EDGE('',*,*,#8656,.F.);
#11449=ORIENTED_EDGE('',*,*,#8657,.T.);
#11450=ORIENTED_EDGE('',*,*,#8658,.T.);
#11451=ORIENTED_EDGE('',*,*,#8527,.T.);
#11452=ORIENTED_EDGE('',*,*,#8659,.F.);
#11453=ORIENTED_EDGE('',*,*,#8660,.T.);
#11454=ORIENTED_EDGE('',*,*,#8661,.T.);
#11455=ORIENTED_EDGE('',*,*,#8525,.T.);
#11456=ORIENTED_EDGE('',*,*,#8662,.F.);
#11457=ORIENTED_EDGE('',*,*,#8663,.T.);
#11458=ORIENTED_EDGE('',*,*,#8664,.T.);
#11459=ORIENTED_EDGE('',*,*,#8540,.T.);
#11460=ORIENTED_EDGE('',*,*,#8665,.F.);
#11461=ORIENTED_EDGE('',*,*,#8666,.T.);
#11462=ORIENTED_EDGE('',*,*,#8667,.T.);
#11463=ORIENTED_EDGE('',*,*,#8536,.T.);
#11464=ORIENTED_EDGE('',*,*,#8668,.F.);
#11465=ORIENTED_EDGE('',*,*,#8669,.T.);
#11466=ORIENTED_EDGE('',*,*,#8670,.T.);
#11467=ORIENTED_EDGE('',*,*,#8534,.T.);
#11468=ORIENTED_EDGE('',*,*,#8671,.F.);
#11469=ORIENTED_EDGE('',*,*,#8672,.T.);
#11470=ORIENTED_EDGE('',*,*,#8673,.T.);
#11471=ORIENTED_EDGE('',*,*,#8543,.T.);
#11472=ORIENTED_EDGE('',*,*,#8674,.F.);
#11473=ORIENTED_EDGE('',*,*,#8675,.T.);
#11474=ORIENTED_EDGE('',*,*,#8676,.T.);
#11475=ORIENTED_EDGE('',*,*,#8546,.T.);
#11476=ORIENTED_EDGE('',*,*,#8677,.F.);
#11477=ORIENTED_EDGE('',*,*,#8678,.T.);
#11478=ORIENTED_EDGE('',*,*,#8679,.T.);
#11479=ORIENTED_EDGE('',*,*,#8680,.T.);
#11480=ORIENTED_EDGE('',*,*,#8681,.F.);
#11481=ORIENTED_EDGE('',*,*,#8682,.T.);
#11482=ORIENTED_EDGE('',*,*,#8683,.T.);
#11483=ORIENTED_EDGE('',*,*,#8617,.T.);
#11484=ORIENTED_EDGE('',*,*,#8684,.F.);
#11485=ORIENTED_EDGE('',*,*,#8685,.T.);
#11486=ORIENTED_EDGE('',*,*,#8686,.T.);
#11487=ORIENTED_EDGE('',*,*,#8615,.T.);
#11488=ORIENTED_EDGE('',*,*,#8687,.F.);
#11489=ORIENTED_EDGE('',*,*,#8688,.T.);
#11490=ORIENTED_EDGE('',*,*,#8689,.T.);
#11491=ORIENTED_EDGE('',*,*,#8621,.T.);
#11492=ORIENTED_EDGE('',*,*,#8690,.F.);
#11493=ORIENTED_EDGE('',*,*,#8691,.T.);
#11494=ORIENTED_EDGE('',*,*,#8692,.T.);
#11495=ORIENTED_EDGE('',*,*,#8624,.T.);
#11496=ORIENTED_EDGE('',*,*,#8693,.F.);
#11497=ORIENTED_EDGE('',*,*,#8694,.T.);
#11498=ORIENTED_EDGE('',*,*,#8695,.T.);
#11499=ORIENTED_EDGE('',*,*,#8633,.T.);
#11500=ORIENTED_EDGE('',*,*,#8696,.F.);
#11501=ORIENTED_EDGE('',*,*,#8697,.T.);
#11502=ORIENTED_EDGE('',*,*,#8698,.T.);
#11503=ORIENTED_EDGE('',*,*,#8629,.T.);
#11504=ORIENTED_EDGE('',*,*,#8699,.F.);
#11505=ORIENTED_EDGE('',*,*,#8700,.T.);
#11506=ORIENTED_EDGE('',*,*,#8701,.T.);
#11507=ORIENTED_EDGE('',*,*,#8627,.T.);
#11508=ORIENTED_EDGE('',*,*,#8702,.F.);
#11509=ORIENTED_EDGE('',*,*,#8703,.T.);
#11510=ORIENTED_EDGE('',*,*,#8704,.T.);
#11511=ORIENTED_EDGE('',*,*,#8638,.T.);
#11512=ORIENTED_EDGE('',*,*,#8705,.F.);
#11513=ORIENTED_EDGE('',*,*,#8706,.T.);
#11514=ORIENTED_EDGE('',*,*,#8707,.T.);
#11515=ORIENTED_EDGE('',*,*,#8636,.T.);
#11516=ORIENTED_EDGE('',*,*,#8708,.F.);
#11517=ORIENTED_EDGE('',*,*,#8709,.T.);
#11518=ORIENTED_EDGE('',*,*,#8710,.T.);
#11519=ORIENTED_EDGE('',*,*,#8642,.T.);
#11520=ORIENTED_EDGE('',*,*,#8711,.F.);
#11521=ORIENTED_EDGE('',*,*,#8712,.T.);
#11522=ORIENTED_EDGE('',*,*,#8713,.T.);
#11523=ORIENTED_EDGE('',*,*,#8645,.T.);
#11524=ORIENTED_EDGE('',*,*,#8714,.F.);
#11525=ORIENTED_EDGE('',*,*,#8715,.T.);
#11526=ORIENTED_EDGE('',*,*,#8716,.T.);
#11527=ORIENTED_EDGE('',*,*,#8584,.T.);
#11528=ORIENTED_EDGE('',*,*,#8717,.F.);
#11529=ORIENTED_EDGE('',*,*,#8718,.T.);
#11530=ORIENTED_EDGE('',*,*,#8719,.T.);
#11531=ORIENTED_EDGE('',*,*,#8582,.T.);
#11532=ORIENTED_EDGE('',*,*,#8720,.F.);
#11533=ORIENTED_EDGE('',*,*,#8721,.T.);
#11534=ORIENTED_EDGE('',*,*,#8722,.T.);
#11535=ORIENTED_EDGE('',*,*,#8588,.T.);
#11536=ORIENTED_EDGE('',*,*,#8723,.F.);
#11537=ORIENTED_EDGE('',*,*,#8724,.T.);
#11538=ORIENTED_EDGE('',*,*,#8725,.T.);
#11539=ORIENTED_EDGE('',*,*,#8591,.T.);
#11540=ORIENTED_EDGE('',*,*,#8726,.F.);
#11541=ORIENTED_EDGE('',*,*,#8727,.T.);
#11542=ORIENTED_EDGE('',*,*,#8728,.T.);
#11543=ORIENTED_EDGE('',*,*,#8600,.T.);
#11544=ORIENTED_EDGE('',*,*,#8729,.F.);
#11545=ORIENTED_EDGE('',*,*,#8730,.T.);
#11546=ORIENTED_EDGE('',*,*,#8731,.T.);
#11547=ORIENTED_EDGE('',*,*,#8596,.T.);
#11548=ORIENTED_EDGE('',*,*,#8732,.F.);
#11549=ORIENTED_EDGE('',*,*,#8733,.T.);
#11550=ORIENTED_EDGE('',*,*,#8734,.T.);
#11551=ORIENTED_EDGE('',*,*,#8594,.T.);
#11552=ORIENTED_EDGE('',*,*,#8735,.F.);
#11553=ORIENTED_EDGE('',*,*,#8736,.T.);
#11554=ORIENTED_EDGE('',*,*,#8737,.T.);
#11555=ORIENTED_EDGE('',*,*,#8605,.T.);
#11556=ORIENTED_EDGE('',*,*,#8738,.F.);
#11557=ORIENTED_EDGE('',*,*,#8739,.T.);
#11558=ORIENTED_EDGE('',*,*,#8740,.T.);
#11559=ORIENTED_EDGE('',*,*,#8603,.T.);
#11560=ORIENTED_EDGE('',*,*,#8741,.F.);
#11561=ORIENTED_EDGE('',*,*,#8742,.T.);
#11562=ORIENTED_EDGE('',*,*,#8743,.T.);
#11563=ORIENTED_EDGE('',*,*,#8609,.T.);
#11564=ORIENTED_EDGE('',*,*,#8744,.F.);
#11565=ORIENTED_EDGE('',*,*,#8745,.T.);
#11566=ORIENTED_EDGE('',*,*,#8746,.T.);
#11567=ORIENTED_EDGE('',*,*,#8612,.T.);
#11568=ORIENTED_EDGE('',*,*,#8747,.F.);
#11569=ORIENTED_EDGE('',*,*,#8748,.T.);
#11570=ORIENTED_EDGE('',*,*,#8749,.T.);
#11571=ORIENTED_EDGE('',*,*,#8551,.T.);
#11572=ORIENTED_EDGE('',*,*,#8750,.F.);
#11573=ORIENTED_EDGE('',*,*,#8751,.T.);
#11574=ORIENTED_EDGE('',*,*,#8752,.T.);
#11575=ORIENTED_EDGE('',*,*,#8549,.T.);
#11576=ORIENTED_EDGE('',*,*,#8753,.F.);
#11577=ORIENTED_EDGE('',*,*,#8754,.T.);
#11578=ORIENTED_EDGE('',*,*,#8755,.T.);
#11579=ORIENTED_EDGE('',*,*,#8555,.T.);
#11580=ORIENTED_EDGE('',*,*,#8756,.F.);
#11581=ORIENTED_EDGE('',*,*,#8757,.T.);
#11582=ORIENTED_EDGE('',*,*,#8758,.T.);
#11583=ORIENTED_EDGE('',*,*,#8558,.T.);
#11584=ORIENTED_EDGE('',*,*,#8759,.F.);
#11585=ORIENTED_EDGE('',*,*,#8760,.T.);
#11586=ORIENTED_EDGE('',*,*,#8761,.T.);
#11587=ORIENTED_EDGE('',*,*,#8566,.T.);
#11588=ORIENTED_EDGE('',*,*,#8762,.F.);
#11589=ORIENTED_EDGE('',*,*,#8763,.T.);
#11590=ORIENTED_EDGE('',*,*,#8764,.T.);
#11591=ORIENTED_EDGE('',*,*,#8563,.T.);
#11592=ORIENTED_EDGE('',*,*,#8765,.F.);
#11593=ORIENTED_EDGE('',*,*,#8766,.T.);
#11594=ORIENTED_EDGE('',*,*,#8767,.T.);
#11595=ORIENTED_EDGE('',*,*,#8561,.T.);
#11596=ORIENTED_EDGE('',*,*,#8768,.F.);
#11597=ORIENTED_EDGE('',*,*,#8769,.T.);
#11598=ORIENTED_EDGE('',*,*,#8770,.T.);
#11599=ORIENTED_EDGE('',*,*,#8576,.T.);
#11600=ORIENTED_EDGE('',*,*,#8771,.F.);
#11601=ORIENTED_EDGE('',*,*,#8772,.T.);
#11602=ORIENTED_EDGE('',*,*,#8773,.T.);
#11603=ORIENTED_EDGE('',*,*,#8572,.T.);
#11604=ORIENTED_EDGE('',*,*,#8774,.F.);
#11605=ORIENTED_EDGE('',*,*,#8775,.T.);
#11606=ORIENTED_EDGE('',*,*,#8776,.T.);
#11607=ORIENTED_EDGE('',*,*,#8570,.T.);
#11608=ORIENTED_EDGE('',*,*,#8777,.F.);
#11609=ORIENTED_EDGE('',*,*,#8778,.T.);
#11610=ORIENTED_EDGE('',*,*,#8779,.T.);
#11611=ORIENTED_EDGE('',*,*,#8579,.T.);
#11612=ORIENTED_EDGE('',*,*,#8780,.F.);
#11613=ORIENTED_EDGE('',*,*,#8781,.T.);
#11614=ORIENTED_EDGE('',*,*,#8782,.T.);
#11615=ORIENTED_EDGE('',*,*,#8515,.T.);
#11616=ORIENTED_EDGE('',*,*,#8783,.F.);
#11617=ORIENTED_EDGE('',*,*,#8784,.T.);
#11618=ORIENTED_EDGE('',*,*,#8785,.F.);
#11619=ORIENTED_EDGE('',*,*,#8786,.F.);
#11620=ORIENTED_EDGE('',*,*,#8465,.T.);
#11621=ORIENTED_EDGE('',*,*,#8787,.F.);
#11622=ORIENTED_EDGE('',*,*,#8680,.F.);
#11623=ORIENTED_EDGE('',*,*,#8618,.T.);
#11624=ORIENTED_EDGE('',*,*,#8683,.F.);
#11625=ORIENTED_EDGE('',*,*,#8788,.F.);
#11626=ORIENTED_EDGE('',*,*,#8462,.T.);
#11627=ORIENTED_EDGE('',*,*,#8787,.T.);
#11628=ORIENTED_EDGE('',*,*,#8464,.T.);
#11629=ORIENTED_EDGE('',*,*,#8789,.T.);
#11630=ORIENTED_EDGE('',*,*,#8681,.T.);
#11631=ORIENTED_EDGE('',*,*,#8682,.F.);
#11632=ORIENTED_EDGE('',*,*,#8789,.F.);
#11633=ORIENTED_EDGE('',*,*,#8463,.T.);
#11634=ORIENTED_EDGE('',*,*,#8788,.T.);
#11635=ORIENTED_EDGE('',*,*,#8786,.T.);
#11636=ORIENTED_EDGE('',*,*,#8679,.F.);
#11637=ORIENTED_EDGE('',*,*,#8790,.F.);
#11638=ORIENTED_EDGE('',*,*,#8466,.T.);
#11639=ORIENTED_EDGE('',*,*,#8545,.T.);
#11640=ORIENTED_EDGE('',*,*,#8468,.T.);
#11641=ORIENTED_EDGE('',*,*,#8791,.T.);
#11642=ORIENTED_EDGE('',*,*,#8677,.T.);
#11643=ORIENTED_EDGE('',*,*,#8678,.F.);
#11644=ORIENTED_EDGE('',*,*,#8791,.F.);
#11645=ORIENTED_EDGE('',*,*,#8467,.T.);
#11646=ORIENTED_EDGE('',*,*,#8790,.T.);
#11647=ORIENTED_EDGE('',*,*,#8585,.T.);
#11648=ORIENTED_EDGE('',*,*,#8716,.F.);
#11649=ORIENTED_EDGE('',*,*,#8792,.F.);
#11650=ORIENTED_EDGE('',*,*,#8418,.T.);
#11651=ORIENTED_EDGE('',*,*,#8644,.T.);
#11652=ORIENTED_EDGE('',*,*,#8420,.T.);
#11653=ORIENTED_EDGE('',*,*,#8793,.T.);
#11654=ORIENTED_EDGE('',*,*,#8714,.T.);
#11655=ORIENTED_EDGE('',*,*,#8715,.F.);
#11656=ORIENTED_EDGE('',*,*,#8793,.F.);
#11657=ORIENTED_EDGE('',*,*,#8419,.T.);
#11658=ORIENTED_EDGE('',*,*,#8792,.T.);
#11659=ORIENTED_EDGE('',*,*,#8643,.T.);
#11660=ORIENTED_EDGE('',*,*,#8713,.F.);
#11661=ORIENTED_EDGE('',*,*,#8794,.F.);
#11662=ORIENTED_EDGE('',*,*,#8422,.T.);
#11663=ORIENTED_EDGE('',*,*,#8641,.T.);
#11664=ORIENTED_EDGE('',*,*,#8424,.T.);
#11665=ORIENTED_EDGE('',*,*,#8795,.T.);
#11666=ORIENTED_EDGE('',*,*,#8711,.T.);
#11667=ORIENTED_EDGE('',*,*,#8712,.F.);
#11668=ORIENTED_EDGE('',*,*,#8795,.F.);
#11669=ORIENTED_EDGE('',*,*,#8423,.T.);
#11670=ORIENTED_EDGE('',*,*,#8794,.T.);
#11671=ORIENTED_EDGE('',*,*,#8640,.T.);
#11672=ORIENTED_EDGE('',*,*,#8710,.F.);
#11673=ORIENTED_EDGE('',*,*,#8796,.F.);
#11674=ORIENTED_EDGE('',*,*,#8426,.T.);
#11675=ORIENTED_EDGE('',*,*,#8635,.T.);
#11676=ORIENTED_EDGE('',*,*,#8428,.T.);
#11677=ORIENTED_EDGE('',*,*,#8797,.T.);
#11678=ORIENTED_EDGE('',*,*,#8708,.T.);
#11679=ORIENTED_EDGE('',*,*,#8709,.F.);
#11680=ORIENTED_EDGE('',*,*,#8797,.F.);
#11681=ORIENTED_EDGE('',*,*,#8427,.T.);
#11682=ORIENTED_EDGE('',*,*,#8796,.T.);
#11683=ORIENTED_EDGE('',*,*,#8639,.T.);
#11684=ORIENTED_EDGE('',*,*,#8704,.F.);
#11685=ORIENTED_EDGE('',*,*,#8798,.F.);
#11686=ORIENTED_EDGE('',*,*,#8434,.T.);
#11687=ORIENTED_EDGE('',*,*,#8626,.T.);
#11688=ORIENTED_EDGE('',*,*,#8436,.T.);
#11689=ORIENTED_EDGE('',*,*,#8799,.T.);
#11690=ORIENTED_EDGE('',*,*,#8702,.T.);
#11691=ORIENTED_EDGE('',*,*,#8703,.F.);
#11692=ORIENTED_EDGE('',*,*,#8799,.F.);
#11693=ORIENTED_EDGE('',*,*,#8435,.T.);
#11694=ORIENTED_EDGE('',*,*,#8798,.T.);
#11695=ORIENTED_EDGE('',*,*,#8634,.T.);
#11696=ORIENTED_EDGE('',*,*,#8707,.F.);
#11697=ORIENTED_EDGE('',*,*,#8800,.F.);
#11698=ORIENTED_EDGE('',*,*,#8430,.T.);
#11699=ORIENTED_EDGE('',*,*,#8637,.T.);
#11700=ORIENTED_EDGE('',*,*,#8432,.T.);
#11701=ORIENTED_EDGE('',*,*,#8801,.T.);
#11702=ORIENTED_EDGE('',*,*,#8705,.T.);
#11703=ORIENTED_EDGE('',*,*,#8706,.F.);
#11704=ORIENTED_EDGE('',*,*,#8801,.F.);
#11705=ORIENTED_EDGE('',*,*,#8431,.T.);
#11706=ORIENTED_EDGE('',*,*,#8800,.T.);
#11707=ORIENTED_EDGE('',*,*,#8630,.T.);
#11708=ORIENTED_EDGE('',*,*,#8698,.F.);
#11709=ORIENTED_EDGE('',*,*,#8802,.F.);
#11710=ORIENTED_EDGE('',*,*,#8442,.T.);
#11711=ORIENTED_EDGE('',*,*,#8632,.T.);
#11712=ORIENTED_EDGE('',*,*,#8444,.T.);
#11713=ORIENTED_EDGE('',*,*,#8803,.T.);
#11714=ORIENTED_EDGE('',*,*,#8696,.T.);
#11715=ORIENTED_EDGE('',*,*,#8697,.F.);
#11716=ORIENTED_EDGE('',*,*,#8803,.F.);
#11717=ORIENTED_EDGE('',*,*,#8443,.T.);
#11718=ORIENTED_EDGE('',*,*,#8802,.T.);
#11719=ORIENTED_EDGE('',*,*,#8631,.T.);
#11720=ORIENTED_EDGE('',*,*,#8695,.F.);
#11721=ORIENTED_EDGE('',*,*,#8804,.F.);
#11722=ORIENTED_EDGE('',*,*,#8446,.T.);
#11723=ORIENTED_EDGE('',*,*,#8623,.T.);
#11724=ORIENTED_EDGE('',*,*,#8448,.T.);
#11725=ORIENTED_EDGE('',*,*,#8805,.T.);
#11726=ORIENTED_EDGE('',*,*,#8693,.T.);
#11727=ORIENTED_EDGE('',*,*,#8694,.F.);
#11728=ORIENTED_EDGE('',*,*,#8805,.F.);
#11729=ORIENTED_EDGE('',*,*,#8447,.T.);
#11730=ORIENTED_EDGE('',*,*,#8804,.T.);
#11731=ORIENTED_EDGE('',*,*,#8625,.T.);
#11732=ORIENTED_EDGE('',*,*,#8701,.F.);
#11733=ORIENTED_EDGE('',*,*,#8806,.F.);
#11734=ORIENTED_EDGE('',*,*,#8438,.T.);
#11735=ORIENTED_EDGE('',*,*,#8628,.T.);
#11736=ORIENTED_EDGE('',*,*,#8440,.T.);
#11737=ORIENTED_EDGE('',*,*,#8807,.T.);
#11738=ORIENTED_EDGE('',*,*,#8699,.T.);
#11739=ORIENTED_EDGE('',*,*,#8700,.F.);
#11740=ORIENTED_EDGE('',*,*,#8807,.F.);
#11741=ORIENTED_EDGE('',*,*,#8439,.T.);
#11742=ORIENTED_EDGE('',*,*,#8806,.T.);
#11743=ORIENTED_EDGE('',*,*,#8622,.T.);
#11744=ORIENTED_EDGE('',*,*,#8692,.F.);
#11745=ORIENTED_EDGE('',*,*,#8808,.F.);
#11746=ORIENTED_EDGE('',*,*,#8450,.T.);
#11747=ORIENTED_EDGE('',*,*,#8620,.T.);
#11748=ORIENTED_EDGE('',*,*,#8452,.T.);
#11749=ORIENTED_EDGE('',*,*,#8809,.T.);
#11750=ORIENTED_EDGE('',*,*,#8690,.T.);
#11751=ORIENTED_EDGE('',*,*,#8691,.F.);
#11752=ORIENTED_EDGE('',*,*,#8809,.F.);
#11753=ORIENTED_EDGE('',*,*,#8451,.T.);
#11754=ORIENTED_EDGE('',*,*,#8808,.T.);
#11755=ORIENTED_EDGE('',*,*,#8619,.T.);
#11756=ORIENTED_EDGE('',*,*,#8689,.F.);
#11757=ORIENTED_EDGE('',*,*,#8810,.F.);
#11758=ORIENTED_EDGE('',*,*,#8454,.T.);
#11759=ORIENTED_EDGE('',*,*,#8614,.T.);
#11760=ORIENTED_EDGE('',*,*,#8456,.T.);
#11761=ORIENTED_EDGE('',*,*,#8811,.T.);
#11762=ORIENTED_EDGE('',*,*,#8687,.T.);
#11763=ORIENTED_EDGE('',*,*,#8688,.F.);
#11764=ORIENTED_EDGE('',*,*,#8811,.F.);
#11765=ORIENTED_EDGE('',*,*,#8455,.T.);
#11766=ORIENTED_EDGE('',*,*,#8810,.T.);
#11767=ORIENTED_EDGE('',*,*,#8613,.T.);
#11768=ORIENTED_EDGE('',*,*,#8686,.F.);
#11769=ORIENTED_EDGE('',*,*,#8812,.F.);
#11770=ORIENTED_EDGE('',*,*,#8458,.T.);
#11771=ORIENTED_EDGE('',*,*,#8616,.T.);
#11772=ORIENTED_EDGE('',*,*,#8460,.T.);
#11773=ORIENTED_EDGE('',*,*,#8813,.T.);
#11774=ORIENTED_EDGE('',*,*,#8684,.T.);
#11775=ORIENTED_EDGE('',*,*,#8685,.F.);
#11776=ORIENTED_EDGE('',*,*,#8813,.F.);
#11777=ORIENTED_EDGE('',*,*,#8459,.T.);
#11778=ORIENTED_EDGE('',*,*,#8812,.T.);
#11779=ORIENTED_EDGE('',*,*,#8552,.T.);
#11780=ORIENTED_EDGE('',*,*,#8749,.F.);
#11781=ORIENTED_EDGE('',*,*,#8814,.F.);
#11782=ORIENTED_EDGE('',*,*,#8374,.T.);
#11783=ORIENTED_EDGE('',*,*,#8611,.T.);
#11784=ORIENTED_EDGE('',*,*,#8376,.T.);
#11785=ORIENTED_EDGE('',*,*,#8815,.T.);
#11786=ORIENTED_EDGE('',*,*,#8747,.T.);
#11787=ORIENTED_EDGE('',*,*,#8748,.F.);
#11788=ORIENTED_EDGE('',*,*,#8815,.F.);
#11789=ORIENTED_EDGE('',*,*,#8375,.T.);
#11790=ORIENTED_EDGE('',*,*,#8814,.T.);
#11791=ORIENTED_EDGE('',*,*,#8610,.T.);
#11792=ORIENTED_EDGE('',*,*,#8746,.F.);
#11793=ORIENTED_EDGE('',*,*,#8816,.F.);
#11794=ORIENTED_EDGE('',*,*,#8378,.T.);
#11795=ORIENTED_EDGE('',*,*,#8608,.T.);
#11796=ORIENTED_EDGE('',*,*,#8380,.T.);
#11797=ORIENTED_EDGE('',*,*,#8817,.T.);
#11798=ORIENTED_EDGE('',*,*,#8744,.T.);
#11799=ORIENTED_EDGE('',*,*,#8745,.F.);
#11800=ORIENTED_EDGE('',*,*,#8817,.F.);
#11801=ORIENTED_EDGE('',*,*,#8379,.T.);
#11802=ORIENTED_EDGE('',*,*,#8816,.T.);
#11803=ORIENTED_EDGE('',*,*,#8607,.T.);
#11804=ORIENTED_EDGE('',*,*,#8743,.F.);
#11805=ORIENTED_EDGE('',*,*,#8818,.F.);
#11806=ORIENTED_EDGE('',*,*,#8382,.T.);
#11807=ORIENTED_EDGE('',*,*,#8602,.T.);
#11808=ORIENTED_EDGE('',*,*,#8384,.T.);
#11809=ORIENTED_EDGE('',*,*,#8819,.T.);
#11810=ORIENTED_EDGE('',*,*,#8741,.T.);
#11811=ORIENTED_EDGE('',*,*,#8742,.F.);
#11812=ORIENTED_EDGE('',*,*,#8819,.F.);
#11813=ORIENTED_EDGE('',*,*,#8383,.T.);
#11814=ORIENTED_EDGE('',*,*,#8818,.T.);
#11815=ORIENTED_EDGE('',*,*,#8606,.T.);
#11816=ORIENTED_EDGE('',*,*,#8737,.F.);
#11817=ORIENTED_EDGE('',*,*,#8820,.F.);
#11818=ORIENTED_EDGE('',*,*,#8390,.T.);
#11819=ORIENTED_EDGE('',*,*,#8593,.T.);
#11820=ORIENTED_EDGE('',*,*,#8392,.T.);
#11821=ORIENTED_EDGE('',*,*,#8821,.T.);
#11822=ORIENTED_EDGE('',*,*,#8735,.T.);
#11823=ORIENTED_EDGE('',*,*,#8736,.F.);
#11824=ORIENTED_EDGE('',*,*,#8821,.F.);
#11825=ORIENTED_EDGE('',*,*,#8391,.T.);
#11826=ORIENTED_EDGE('',*,*,#8820,.T.);
#11827=ORIENTED_EDGE('',*,*,#8601,.T.);
#11828=ORIENTED_EDGE('',*,*,#8740,.F.);
#11829=ORIENTED_EDGE('',*,*,#8822,.F.);
#11830=ORIENTED_EDGE('',*,*,#8386,.T.);
#11831=ORIENTED_EDGE('',*,*,#8604,.T.);
#11832=ORIENTED_EDGE('',*,*,#8388,.T.);
#11833=ORIENTED_EDGE('',*,*,#8823,.T.);
#11834=ORIENTED_EDGE('',*,*,#8738,.T.);
#11835=ORIENTED_EDGE('',*,*,#8739,.F.);
#11836=ORIENTED_EDGE('',*,*,#8823,.F.);
#11837=ORIENTED_EDGE('',*,*,#8387,.T.);
#11838=ORIENTED_EDGE('',*,*,#8822,.T.);
#11839=ORIENTED_EDGE('',*,*,#8597,.T.);
#11840=ORIENTED_EDGE('',*,*,#8731,.F.);
#11841=ORIENTED_EDGE('',*,*,#8824,.F.);
#11842=ORIENTED_EDGE('',*,*,#8398,.T.);
#11843=ORIENTED_EDGE('',*,*,#8599,.T.);
#11844=ORIENTED_EDGE('',*,*,#8400,.T.);
#11845=ORIENTED_EDGE('',*,*,#8825,.T.);
#11846=ORIENTED_EDGE('',*,*,#8729,.T.);
#11847=ORIENTED_EDGE('',*,*,#8730,.F.);
#11848=ORIENTED_EDGE('',*,*,#8825,.F.);
#11849=ORIENTED_EDGE('',*,*,#8399,.T.);
#11850=ORIENTED_EDGE('',*,*,#8824,.T.);
#11851=ORIENTED_EDGE('',*,*,#8598,.T.);
#11852=ORIENTED_EDGE('',*,*,#8728,.F.);
#11853=ORIENTED_EDGE('',*,*,#8826,.F.);
#11854=ORIENTED_EDGE('',*,*,#8402,.T.);
#11855=ORIENTED_EDGE('',*,*,#8590,.T.);
#11856=ORIENTED_EDGE('',*,*,#8404,.T.);
#11857=ORIENTED_EDGE('',*,*,#8827,.T.);
#11858=ORIENTED_EDGE('',*,*,#8726,.T.);
#11859=ORIENTED_EDGE('',*,*,#8727,.F.);
#11860=ORIENTED_EDGE('',*,*,#8827,.F.);
#11861=ORIENTED_EDGE('',*,*,#8403,.T.);
#11862=ORIENTED_EDGE('',*,*,#8826,.T.);
#11863=ORIENTED_EDGE('',*,*,#8592,.T.);
#11864=ORIENTED_EDGE('',*,*,#8734,.F.);
#11865=ORIENTED_EDGE('',*,*,#8828,.F.);
#11866=ORIENTED_EDGE('',*,*,#8394,.T.);
#11867=ORIENTED_EDGE('',*,*,#8595,.T.);
#11868=ORIENTED_EDGE('',*,*,#8396,.T.);
#11869=ORIENTED_EDGE('',*,*,#8829,.T.);
#11870=ORIENTED_EDGE('',*,*,#8732,.T.);
#11871=ORIENTED_EDGE('',*,*,#8733,.F.);
#11872=ORIENTED_EDGE('',*,*,#8829,.F.);
#11873=ORIENTED_EDGE('',*,*,#8395,.T.);
#11874=ORIENTED_EDGE('',*,*,#8828,.T.);
#11875=ORIENTED_EDGE('',*,*,#8589,.T.);
#11876=ORIENTED_EDGE('',*,*,#8725,.F.);
#11877=ORIENTED_EDGE('',*,*,#8830,.F.);
#11878=ORIENTED_EDGE('',*,*,#8406,.T.);
#11879=ORIENTED_EDGE('',*,*,#8587,.T.);
#11880=ORIENTED_EDGE('',*,*,#8408,.T.);
#11881=ORIENTED_EDGE('',*,*,#8831,.T.);
#11882=ORIENTED_EDGE('',*,*,#8723,.T.);
#11883=ORIENTED_EDGE('',*,*,#8724,.F.);
#11884=ORIENTED_EDGE('',*,*,#8831,.F.);
#11885=ORIENTED_EDGE('',*,*,#8407,.T.);
#11886=ORIENTED_EDGE('',*,*,#8830,.T.);
#11887=ORIENTED_EDGE('',*,*,#8586,.T.);
#11888=ORIENTED_EDGE('',*,*,#8722,.F.);
#11889=ORIENTED_EDGE('',*,*,#8832,.F.);
#11890=ORIENTED_EDGE('',*,*,#8410,.T.);
#11891=ORIENTED_EDGE('',*,*,#8581,.T.);
#11892=ORIENTED_EDGE('',*,*,#8412,.T.);
#11893=ORIENTED_EDGE('',*,*,#8833,.T.);
#11894=ORIENTED_EDGE('',*,*,#8720,.T.);
#11895=ORIENTED_EDGE('',*,*,#8721,.F.);
#11896=ORIENTED_EDGE('',*,*,#8833,.F.);
#11897=ORIENTED_EDGE('',*,*,#8411,.T.);
#11898=ORIENTED_EDGE('',*,*,#8832,.T.);
#11899=ORIENTED_EDGE('',*,*,#8580,.T.);
#11900=ORIENTED_EDGE('',*,*,#8719,.F.);
#11901=ORIENTED_EDGE('',*,*,#8834,.F.);
#11902=ORIENTED_EDGE('',*,*,#8414,.T.);
#11903=ORIENTED_EDGE('',*,*,#8583,.T.);
#11904=ORIENTED_EDGE('',*,*,#8416,.T.);
#11905=ORIENTED_EDGE('',*,*,#8835,.T.);
#11906=ORIENTED_EDGE('',*,*,#8717,.T.);
#11907=ORIENTED_EDGE('',*,*,#8718,.F.);
#11908=ORIENTED_EDGE('',*,*,#8835,.F.);
#11909=ORIENTED_EDGE('',*,*,#8415,.T.);
#11910=ORIENTED_EDGE('',*,*,#8834,.T.);
#11911=ORIENTED_EDGE('',*,*,#8516,.T.);
#11912=ORIENTED_EDGE('',*,*,#8782,.F.);
#11913=ORIENTED_EDGE('',*,*,#8836,.F.);
#11914=ORIENTED_EDGE('',*,*,#8330,.T.);
#11915=ORIENTED_EDGE('',*,*,#8578,.T.);
#11916=ORIENTED_EDGE('',*,*,#8332,.T.);
#11917=ORIENTED_EDGE('',*,*,#8837,.T.);
#11918=ORIENTED_EDGE('',*,*,#8780,.T.);
#11919=ORIENTED_EDGE('',*,*,#8781,.F.);
#11920=ORIENTED_EDGE('',*,*,#8837,.F.);
#11921=ORIENTED_EDGE('',*,*,#8331,.T.);
#11922=ORIENTED_EDGE('',*,*,#8836,.T.);
#11923=ORIENTED_EDGE('',*,*,#8577,.T.);
#11924=ORIENTED_EDGE('',*,*,#8779,.F.);
#11925=ORIENTED_EDGE('',*,*,#8838,.F.);
#11926=ORIENTED_EDGE('',*,*,#8334,.T.);
#11927=ORIENTED_EDGE('',*,*,#8569,.T.);
#11928=ORIENTED_EDGE('',*,*,#8336,.T.);
#11929=ORIENTED_EDGE('',*,*,#8839,.T.);
#11930=ORIENTED_EDGE('',*,*,#8777,.T.);
#11931=ORIENTED_EDGE('',*,*,#8778,.F.);
#11932=ORIENTED_EDGE('',*,*,#8839,.F.);
#11933=ORIENTED_EDGE('',*,*,#8335,.T.);
#11934=ORIENTED_EDGE('',*,*,#8838,.T.);
#11935=ORIENTED_EDGE('',*,*,#8573,.T.);
#11936=ORIENTED_EDGE('',*,*,#8773,.F.);
#11937=ORIENTED_EDGE('',*,*,#8840,.F.);
#11938=ORIENTED_EDGE('',*,*,#8342,.T.);
#11939=ORIENTED_EDGE('',*,*,#8575,.T.);
#11940=ORIENTED_EDGE('',*,*,#8344,.T.);
#11941=ORIENTED_EDGE('',*,*,#8841,.T.);
#11942=ORIENTED_EDGE('',*,*,#8771,.T.);
#11943=ORIENTED_EDGE('',*,*,#8772,.F.);
#11944=ORIENTED_EDGE('',*,*,#8841,.F.);
#11945=ORIENTED_EDGE('',*,*,#8343,.T.);
#11946=ORIENTED_EDGE('',*,*,#8840,.T.);
#11947=ORIENTED_EDGE('',*,*,#8574,.T.);
#11948=ORIENTED_EDGE('',*,*,#8770,.F.);
#11949=ORIENTED_EDGE('',*,*,#8842,.F.);
#11950=ORIENTED_EDGE('',*,*,#8346,.T.);
#11951=ORIENTED_EDGE('',*,*,#8560,.T.);
#11952=ORIENTED_EDGE('',*,*,#8348,.T.);
#11953=ORIENTED_EDGE('',*,*,#8843,.T.);
#11954=ORIENTED_EDGE('',*,*,#8768,.T.);
#11955=ORIENTED_EDGE('',*,*,#8769,.F.);
#11956=ORIENTED_EDGE('',*,*,#8843,.F.);
#11957=ORIENTED_EDGE('',*,*,#8347,.T.);
#11958=ORIENTED_EDGE('',*,*,#8842,.T.);
#11959=ORIENTED_EDGE('',*,*,#8568,.T.);
#11960=ORIENTED_EDGE('',*,*,#8776,.F.);
#11961=ORIENTED_EDGE('',*,*,#8844,.F.);
#11962=ORIENTED_EDGE('',*,*,#8338,.T.);
#11963=ORIENTED_EDGE('',*,*,#8571,.T.);
#11964=ORIENTED_EDGE('',*,*,#8340,.T.);
#11965=ORIENTED_EDGE('',*,*,#8845,.T.);
#11966=ORIENTED_EDGE('',*,*,#8774,.T.);
#11967=ORIENTED_EDGE('',*,*,#8775,.F.);
#11968=ORIENTED_EDGE('',*,*,#8845,.F.);
#11969=ORIENTED_EDGE('',*,*,#8339,.T.);
#11970=ORIENTED_EDGE('',*,*,#8844,.T.);
#11971=ORIENTED_EDGE('',*,*,#8567,.T.);
#11972=ORIENTED_EDGE('',*,*,#8761,.F.);
#11973=ORIENTED_EDGE('',*,*,#8846,.F.);
#11974=ORIENTED_EDGE('',*,*,#8358,.T.);
#11975=ORIENTED_EDGE('',*,*,#8557,.T.);
#11976=ORIENTED_EDGE('',*,*,#8360,.T.);
#11977=ORIENTED_EDGE('',*,*,#8847,.T.);
#11978=ORIENTED_EDGE('',*,*,#8759,.T.);
#11979=ORIENTED_EDGE('',*,*,#8760,.F.);
#11980=ORIENTED_EDGE('',*,*,#8847,.F.);
#11981=ORIENTED_EDGE('',*,*,#8359,.T.);
#11982=ORIENTED_EDGE('',*,*,#8846,.T.);
#11983=ORIENTED_EDGE('',*,*,#8564,.T.);
#11984=ORIENTED_EDGE('',*,*,#8764,.F.);
#11985=ORIENTED_EDGE('',*,*,#8848,.F.);
#11986=ORIENTED_EDGE('',*,*,#8354,.T.);
#11987=ORIENTED_EDGE('',*,*,#8565,.T.);
#11988=ORIENTED_EDGE('',*,*,#8356,.T.);
#11989=ORIENTED_EDGE('',*,*,#8849,.T.);
#11990=ORIENTED_EDGE('',*,*,#8762,.T.);
#11991=ORIENTED_EDGE('',*,*,#8763,.F.);
#11992=ORIENTED_EDGE('',*,*,#8849,.F.);
#11993=ORIENTED_EDGE('',*,*,#8355,.T.);
#11994=ORIENTED_EDGE('',*,*,#8848,.T.);
#11995=ORIENTED_EDGE('',*,*,#8559,.T.);
#11996=ORIENTED_EDGE('',*,*,#8767,.F.);
#11997=ORIENTED_EDGE('',*,*,#8850,.F.);
#11998=ORIENTED_EDGE('',*,*,#8350,.T.);
#11999=ORIENTED_EDGE('',*,*,#8562,.T.);
#12000=ORIENTED_EDGE('',*,*,#8352,.T.);
#12001=ORIENTED_EDGE('',*,*,#8851,.T.);
#12002=ORIENTED_EDGE('',*,*,#8765,.T.);
#12003=ORIENTED_EDGE('',*,*,#8766,.F.);
#12004=ORIENTED_EDGE('',*,*,#8851,.F.);
#12005=ORIENTED_EDGE('',*,*,#8351,.T.);
#12006=ORIENTED_EDGE('',*,*,#8850,.T.);
#12007=ORIENTED_EDGE('',*,*,#8556,.T.);
#12008=ORIENTED_EDGE('',*,*,#8758,.F.);
#12009=ORIENTED_EDGE('',*,*,#8852,.F.);
#12010=ORIENTED_EDGE('',*,*,#8362,.T.);
#12011=ORIENTED_EDGE('',*,*,#8554,.T.);
#12012=ORIENTED_EDGE('',*,*,#8364,.T.);
#12013=ORIENTED_EDGE('',*,*,#8853,.T.);
#12014=ORIENTED_EDGE('',*,*,#8756,.T.);
#12015=ORIENTED_EDGE('',*,*,#8757,.F.);
#12016=ORIENTED_EDGE('',*,*,#8853,.F.);
#12017=ORIENTED_EDGE('',*,*,#8363,.T.);
#12018=ORIENTED_EDGE('',*,*,#8852,.T.);
#12019=ORIENTED_EDGE('',*,*,#8553,.T.);
#12020=ORIENTED_EDGE('',*,*,#8755,.F.);
#12021=ORIENTED_EDGE('',*,*,#8854,.F.);
#12022=ORIENTED_EDGE('',*,*,#8366,.T.);
#12023=ORIENTED_EDGE('',*,*,#8548,.T.);
#12024=ORIENTED_EDGE('',*,*,#8368,.T.);
#12025=ORIENTED_EDGE('',*,*,#8855,.T.);
#12026=ORIENTED_EDGE('',*,*,#8753,.T.);
#12027=ORIENTED_EDGE('',*,*,#8754,.F.);
#12028=ORIENTED_EDGE('',*,*,#8855,.F.);
#12029=ORIENTED_EDGE('',*,*,#8367,.T.);
#12030=ORIENTED_EDGE('',*,*,#8854,.T.);
#12031=ORIENTED_EDGE('',*,*,#8547,.T.);
#12032=ORIENTED_EDGE('',*,*,#8752,.F.);
#12033=ORIENTED_EDGE('',*,*,#8856,.F.);
#12034=ORIENTED_EDGE('',*,*,#8370,.T.);
#12035=ORIENTED_EDGE('',*,*,#8550,.T.);
#12036=ORIENTED_EDGE('',*,*,#8372,.T.);
#12037=ORIENTED_EDGE('',*,*,#8857,.T.);
#12038=ORIENTED_EDGE('',*,*,#8750,.T.);
#12039=ORIENTED_EDGE('',*,*,#8751,.F.);
#12040=ORIENTED_EDGE('',*,*,#8857,.F.);
#12041=ORIENTED_EDGE('',*,*,#8371,.T.);
#12042=ORIENTED_EDGE('',*,*,#8856,.T.);
#12043=ORIENTED_EDGE('',*,*,#8544,.T.);
#12044=ORIENTED_EDGE('',*,*,#8676,.F.);
#12045=ORIENTED_EDGE('',*,*,#8858,.F.);
#12046=ORIENTED_EDGE('',*,*,#8470,.T.);
#12047=ORIENTED_EDGE('',*,*,#8542,.T.);
#12048=ORIENTED_EDGE('',*,*,#8472,.T.);
#12049=ORIENTED_EDGE('',*,*,#8859,.T.);
#12050=ORIENTED_EDGE('',*,*,#8674,.T.);
#12051=ORIENTED_EDGE('',*,*,#8675,.F.);
#12052=ORIENTED_EDGE('',*,*,#8859,.F.);
#12053=ORIENTED_EDGE('',*,*,#8471,.T.);
#12054=ORIENTED_EDGE('',*,*,#8858,.T.);
#12055=ORIENTED_EDGE('',*,*,#8541,.T.);
#12056=ORIENTED_EDGE('',*,*,#8673,.F.);
#12057=ORIENTED_EDGE('',*,*,#8860,.F.);
#12058=ORIENTED_EDGE('',*,*,#8474,.T.);
#12059=ORIENTED_EDGE('',*,*,#8533,.T.);
#12060=ORIENTED_EDGE('',*,*,#8476,.T.);
#12061=ORIENTED_EDGE('',*,*,#8861,.T.);
#12062=ORIENTED_EDGE('',*,*,#8671,.T.);
#12063=ORIENTED_EDGE('',*,*,#8672,.F.);
#12064=ORIENTED_EDGE('',*,*,#8861,.F.);
#12065=ORIENTED_EDGE('',*,*,#8475,.T.);
#12066=ORIENTED_EDGE('',*,*,#8860,.T.);
#12067=ORIENTED_EDGE('',*,*,#8537,.T.);
#12068=ORIENTED_EDGE('',*,*,#8667,.F.);
#12069=ORIENTED_EDGE('',*,*,#8862,.F.);
#12070=ORIENTED_EDGE('',*,*,#8482,.T.);
#12071=ORIENTED_EDGE('',*,*,#8539,.T.);
#12072=ORIENTED_EDGE('',*,*,#8484,.T.);
#12073=ORIENTED_EDGE('',*,*,#8863,.T.);
#12074=ORIENTED_EDGE('',*,*,#8665,.T.);
#12075=ORIENTED_EDGE('',*,*,#8666,.F.);
#12076=ORIENTED_EDGE('',*,*,#8863,.F.);
#12077=ORIENTED_EDGE('',*,*,#8483,.T.);
#12078=ORIENTED_EDGE('',*,*,#8862,.T.);
#12079=ORIENTED_EDGE('',*,*,#8538,.T.);
#12080=ORIENTED_EDGE('',*,*,#8664,.F.);
#12081=ORIENTED_EDGE('',*,*,#8864,.F.);
#12082=ORIENTED_EDGE('',*,*,#8486,.T.);
#12083=ORIENTED_EDGE('',*,*,#8524,.T.);
#12084=ORIENTED_EDGE('',*,*,#8488,.T.);
#12085=ORIENTED_EDGE('',*,*,#8865,.T.);
#12086=ORIENTED_EDGE('',*,*,#8662,.T.);
#12087=ORIENTED_EDGE('',*,*,#8663,.F.);
#12088=ORIENTED_EDGE('',*,*,#8865,.F.);
#12089=ORIENTED_EDGE('',*,*,#8487,.T.);
#12090=ORIENTED_EDGE('',*,*,#8864,.T.);
#12091=ORIENTED_EDGE('',*,*,#8532,.T.);
#12092=ORIENTED_EDGE('',*,*,#8670,.F.);
#12093=ORIENTED_EDGE('',*,*,#8866,.F.);
#12094=ORIENTED_EDGE('',*,*,#8478,.T.);
#12095=ORIENTED_EDGE('',*,*,#8535,.T.);
#12096=ORIENTED_EDGE('',*,*,#8480,.T.);
#12097=ORIENTED_EDGE('',*,*,#8867,.T.);
#12098=ORIENTED_EDGE('',*,*,#8668,.T.);
#12099=ORIENTED_EDGE('',*,*,#8669,.F.);
#12100=ORIENTED_EDGE('',*,*,#8867,.F.);
#12101=ORIENTED_EDGE('',*,*,#8479,.T.);
#12102=ORIENTED_EDGE('',*,*,#8866,.T.);
#12103=ORIENTED_EDGE('',*,*,#8531,.T.);
#12104=ORIENTED_EDGE('',*,*,#8655,.F.);
#12105=ORIENTED_EDGE('',*,*,#8868,.F.);
#12106=ORIENTED_EDGE('',*,*,#8498,.T.);
#12107=ORIENTED_EDGE('',*,*,#8521,.T.);
#12108=ORIENTED_EDGE('',*,*,#8500,.T.);
#12109=ORIENTED_EDGE('',*,*,#8869,.T.);
#12110=ORIENTED_EDGE('',*,*,#8653,.T.);
#12111=ORIENTED_EDGE('',*,*,#8654,.F.);
#12112=ORIENTED_EDGE('',*,*,#8869,.F.);
#12113=ORIENTED_EDGE('',*,*,#8499,.T.);
#12114=ORIENTED_EDGE('',*,*,#8868,.T.);
#12115=ORIENTED_EDGE('',*,*,#8528,.T.);
#12116=ORIENTED_EDGE('',*,*,#8658,.F.);
#12117=ORIENTED_EDGE('',*,*,#8870,.F.);
#12118=ORIENTED_EDGE('',*,*,#8494,.T.);
#12119=ORIENTED_EDGE('',*,*,#8529,.T.);
#12120=ORIENTED_EDGE('',*,*,#8496,.T.);
#12121=ORIENTED_EDGE('',*,*,#8871,.T.);
#12122=ORIENTED_EDGE('',*,*,#8656,.T.);
#12123=ORIENTED_EDGE('',*,*,#8657,.F.);
#12124=ORIENTED_EDGE('',*,*,#8871,.F.);
#12125=ORIENTED_EDGE('',*,*,#8495,.T.);
#12126=ORIENTED_EDGE('',*,*,#8870,.T.);
#12127=ORIENTED_EDGE('',*,*,#8523,.T.);
#12128=ORIENTED_EDGE('',*,*,#8661,.F.);
#12129=ORIENTED_EDGE('',*,*,#8872,.F.);
#12130=ORIENTED_EDGE('',*,*,#8490,.T.);
#12131=ORIENTED_EDGE('',*,*,#8526,.T.);
#12132=ORIENTED_EDGE('',*,*,#8492,.T.);
#12133=ORIENTED_EDGE('',*,*,#8873,.T.);
#12134=ORIENTED_EDGE('',*,*,#8659,.T.);
#12135=ORIENTED_EDGE('',*,*,#8660,.F.);
#12136=ORIENTED_EDGE('',*,*,#8873,.F.);
#12137=ORIENTED_EDGE('',*,*,#8491,.T.);
#12138=ORIENTED_EDGE('',*,*,#8872,.T.);
#12139=ORIENTED_EDGE('',*,*,#8520,.T.);
#12140=ORIENTED_EDGE('',*,*,#8652,.F.);
#12141=ORIENTED_EDGE('',*,*,#8874,.F.);
#12142=ORIENTED_EDGE('',*,*,#8502,.T.);
#12143=ORIENTED_EDGE('',*,*,#8518,.T.);
#12144=ORIENTED_EDGE('',*,*,#8504,.T.);
#12145=ORIENTED_EDGE('',*,*,#8875,.T.);
#12146=ORIENTED_EDGE('',*,*,#8650,.T.);
#12147=ORIENTED_EDGE('',*,*,#8651,.F.);
#12148=ORIENTED_EDGE('',*,*,#8875,.F.);
#12149=ORIENTED_EDGE('',*,*,#8503,.T.);
#12150=ORIENTED_EDGE('',*,*,#8874,.T.);
#12151=ORIENTED_EDGE('',*,*,#8517,.T.);
#12152=ORIENTED_EDGE('',*,*,#8649,.F.);
#12153=ORIENTED_EDGE('',*,*,#8876,.F.);
#12154=ORIENTED_EDGE('',*,*,#8506,.T.);
#12155=ORIENTED_EDGE('',*,*,#8512,.T.);
#12156=ORIENTED_EDGE('',*,*,#8508,.T.);
#12157=ORIENTED_EDGE('',*,*,#8877,.T.);
#12158=ORIENTED_EDGE('',*,*,#8647,.T.);
#12159=ORIENTED_EDGE('',*,*,#8648,.F.);
#12160=ORIENTED_EDGE('',*,*,#8877,.F.);
#12161=ORIENTED_EDGE('',*,*,#8507,.T.);
#12162=ORIENTED_EDGE('',*,*,#8876,.T.);
#12163=ORIENTED_EDGE('',*,*,#8511,.T.);
#12164=ORIENTED_EDGE('',*,*,#8646,.F.);
#12165=ORIENTED_EDGE('',*,*,#8878,.F.);
#12166=ORIENTED_EDGE('',*,*,#8326,.T.);
#12167=ORIENTED_EDGE('',*,*,#8514,.T.);
#12168=ORIENTED_EDGE('',*,*,#8328,.T.);
#12169=ORIENTED_EDGE('',*,*,#8879,.T.);
#12170=ORIENTED_EDGE('',*,*,#8783,.T.);
#12171=ORIENTED_EDGE('',*,*,#8784,.F.);
#12172=ORIENTED_EDGE('',*,*,#8879,.F.);
#12173=ORIENTED_EDGE('',*,*,#8327,.T.);
#12174=ORIENTED_EDGE('',*,*,#8878,.T.);
#12175=ORIENTED_EDGE('',*,*,#8510,.T.);
#12176=ORIENTED_EDGE('',*,*,#8880,.T.);
#12177=ORIENTED_EDGE('',*,*,#8785,.T.);
#12178=ORIENTED_EDGE('',*,*,#8880,.F.);
#16555=PLANE('',#17837);
#16556=PLANE('',#18113);
#16660=ADVANCED_FACE('',(#3544,#3477),#16555,.F.);
#16661=ADVANCED_FACE('',(#3545),#3001,.T.);
#16662=ADVANCED_FACE('',(#3546),#3002,.T.);
#16663=ADVANCED_FACE('',(#3547),#3003,.T.);
#16664=ADVANCED_FACE('',(#3548),#3004,.T.);
#16665=ADVANCED_FACE('',(#3549),#3005,.T.);
#16666=ADVANCED_FACE('',(#3550),#3006,.T.);
#16667=ADVANCED_FACE('',(#3551),#3007,.T.);
#16668=ADVANCED_FACE('',(#3552),#3008,.T.);
#16669=ADVANCED_FACE('',(#3553),#3009,.T.);
#16670=ADVANCED_FACE('',(#3554),#3010,.T.);
#16671=ADVANCED_FACE('',(#3555),#3011,.T.);
#16672=ADVANCED_FACE('',(#3556),#3012,.T.);
#16673=ADVANCED_FACE('',(#3557),#3013,.T.);
#16674=ADVANCED_FACE('',(#3558),#3014,.T.);
#16675=ADVANCED_FACE('',(#3559),#3015,.T.);
#16676=ADVANCED_FACE('',(#3560),#3016,.T.);
#16677=ADVANCED_FACE('',(#3561),#3017,.T.);
#16678=ADVANCED_FACE('',(#3562),#3018,.T.);
#16679=ADVANCED_FACE('',(#3563),#3019,.T.);
#16680=ADVANCED_FACE('',(#3564),#3020,.T.);
#16681=ADVANCED_FACE('',(#3565),#3021,.T.);
#16682=ADVANCED_FACE('',(#3566),#3022,.T.);
#16683=ADVANCED_FACE('',(#3567),#3023,.T.);
#16684=ADVANCED_FACE('',(#3568),#3024,.T.);
#16685=ADVANCED_FACE('',(#3569),#3025,.T.);
#16686=ADVANCED_FACE('',(#3570),#3026,.T.);
#16687=ADVANCED_FACE('',(#3571),#3027,.T.);
#16688=ADVANCED_FACE('',(#3572),#3028,.T.);
#16689=ADVANCED_FACE('',(#3573),#3029,.T.);
#16690=ADVANCED_FACE('',(#3574),#3030,.T.);
#16691=ADVANCED_FACE('',(#3575),#3031,.T.);
#16692=ADVANCED_FACE('',(#3576),#3032,.T.);
#16693=ADVANCED_FACE('',(#3577),#3033,.T.);
#16694=ADVANCED_FACE('',(#3578),#3034,.T.);
#16695=ADVANCED_FACE('',(#3579),#3035,.T.);
#16696=ADVANCED_FACE('',(#3580),#3036,.T.);
#16697=ADVANCED_FACE('',(#3581),#3037,.T.);
#16698=ADVANCED_FACE('',(#3582),#3038,.T.);
#16699=ADVANCED_FACE('',(#3583),#3039,.T.);
#16700=ADVANCED_FACE('',(#3584),#3040,.T.);
#16701=ADVANCED_FACE('',(#3585),#3041,.T.);
#16702=ADVANCED_FACE('',(#3586),#3042,.T.);
#16703=ADVANCED_FACE('',(#3587),#3043,.T.);
#16704=ADVANCED_FACE('',(#3588),#3044,.T.);
#16705=ADVANCED_FACE('',(#3589),#3045,.T.);
#16706=ADVANCED_FACE('',(#3590,#3478),#16556,.F.);
#16707=ADVANCED_FACE('',(#3591),#3046,.T.);
#16708=ADVANCED_FACE('',(#3592),#3047,.T.);
#16709=ADVANCED_FACE('',(#3593),#3048,.T.);
#16710=ADVANCED_FACE('',(#3594),#3049,.T.);
#16711=ADVANCED_FACE('',(#3595),#3050,.T.);
#16712=ADVANCED_FACE('',(#3596),#3051,.T.);
#16713=ADVANCED_FACE('',(#3597),#3052,.T.);
#16714=ADVANCED_FACE('',(#3598),#3053,.T.);
#16715=ADVANCED_FACE('',(#3599),#3054,.T.);
#16716=ADVANCED_FACE('',(#3600),#3055,.T.);
#16717=ADVANCED_FACE('',(#3601),#3056,.T.);
#16718=ADVANCED_FACE('',(#3602),#3057,.T.);
#16719=ADVANCED_FACE('',(#3603),#3058,.T.);
#16720=ADVANCED_FACE('',(#3604),#3059,.T.);
#16721=ADVANCED_FACE('',(#3605),#3060,.T.);
#16722=ADVANCED_FACE('',(#3606),#3061,.T.);
#16723=ADVANCED_FACE('',(#3607),#3062,.T.);
#16724=ADVANCED_FACE('',(#3608),#3063,.T.);
#16725=ADVANCED_FACE('',(#3609),#3064,.T.);
#16726=ADVANCED_FACE('',(#3610),#3065,.T.);
#16727=ADVANCED_FACE('',(#3611),#3066,.T.);
#16728=ADVANCED_FACE('',(#3612),#3067,.T.);
#16729=ADVANCED_FACE('',(#3613),#3068,.T.);
#16730=ADVANCED_FACE('',(#3614),#3069,.T.);
#16731=ADVANCED_FACE('',(#3615),#3070,.T.);
#16732=ADVANCED_FACE('',(#3616),#3071,.T.);
#16733=ADVANCED_FACE('',(#3617),#3072,.T.);
#16734=ADVANCED_FACE('',(#3618),#3073,.T.);
#16735=ADVANCED_FACE('',(#3619),#3074,.T.);
#16736=ADVANCED_FACE('',(#3620),#3075,.T.);
#16737=ADVANCED_FACE('',(#3621),#3076,.T.);
#16738=ADVANCED_FACE('',(#3622),#3077,.T.);
#16739=ADVANCED_FACE('',(#3623),#3078,.T.);
#16740=ADVANCED_FACE('',(#3624),#3079,.T.);
#16741=ADVANCED_FACE('',(#3625),#3080,.T.);
#16742=ADVANCED_FACE('',(#3626),#3081,.T.);
#16743=ADVANCED_FACE('',(#3627),#3082,.T.);
#16744=ADVANCED_FACE('',(#3628),#3083,.T.);
#16745=ADVANCED_FACE('',(#3629),#3084,.T.);
#16746=ADVANCED_FACE('',(#3630),#3085,.T.);
#16747=ADVANCED_FACE('',(#3631),#3086,.T.);
#16748=ADVANCED_FACE('',(#3632),#3087,.T.);
#16749=ADVANCED_FACE('',(#3633),#3088,.T.);
#16750=ADVANCED_FACE('',(#3634),#3089,.T.);
#16751=ADVANCED_FACE('',(#3635),#3090,.T.);
#16752=ADVANCED_FACE('',(#3636),#3091,.T.);
#16753=ADVANCED_FACE('',(#3637),#3092,.T.);
#16754=ADVANCED_FACE('',(#3638),#3093,.T.);
#16755=ADVANCED_FACE('',(#3639),#3094,.T.);
#16756=ADVANCED_FACE('',(#3640),#3095,.T.);
#16757=ADVANCED_FACE('',(#3641),#3096,.T.);
#16758=ADVANCED_FACE('',(#3642),#3097,.T.);
#16759=ADVANCED_FACE('',(#3643),#3098,.T.);
#16760=ADVANCED_FACE('',(#3644),#3099,.T.);
#16761=ADVANCED_FACE('',(#3645),#3100,.T.);
#16762=ADVANCED_FACE('',(#3646),#3101,.T.);
#16763=ADVANCED_FACE('',(#3647),#3102,.T.);
#16764=ADVANCED_FACE('',(#3648),#3103,.T.);
#16765=ADVANCED_FACE('',(#3649),#3104,.T.);
#16766=ADVANCED_FACE('',(#3650),#3105,.T.);
#16767=ADVANCED_FACE('',(#3651),#3106,.T.);
#16768=ADVANCED_FACE('',(#3652),#3107,.T.);
#16769=ADVANCED_FACE('',(#3653),#3108,.T.);
#16770=ADVANCED_FACE('',(#3654),#3109,.T.);
#16771=ADVANCED_FACE('',(#3655),#3110,.T.);
#16772=ADVANCED_FACE('',(#3656),#3111,.T.);
#16773=ADVANCED_FACE('',(#3657),#3112,.T.);
#16774=ADVANCED_FACE('',(#3658),#3113,.T.);
#16775=ADVANCED_FACE('',(#3659),#3114,.T.);
#16776=ADVANCED_FACE('',(#3660),#3115,.T.);
#16777=ADVANCED_FACE('',(#3661),#3116,.T.);
#16778=ADVANCED_FACE('',(#3662),#3117,.T.);
#16779=ADVANCED_FACE('',(#3663),#3118,.T.);
#16780=ADVANCED_FACE('',(#3664),#3119,.T.);
#16781=ADVANCED_FACE('',(#3665),#3120,.T.);
#16782=ADVANCED_FACE('',(#3666),#3121,.T.);
#16783=ADVANCED_FACE('',(#3667),#3122,.T.);
#16784=ADVANCED_FACE('',(#3668),#3123,.T.);
#16785=ADVANCED_FACE('',(#3669),#3124,.T.);
#16786=ADVANCED_FACE('',(#3670),#3125,.T.);
#16787=ADVANCED_FACE('',(#3671),#3126,.T.);
#16788=ADVANCED_FACE('',(#3672),#3127,.T.);
#16789=ADVANCED_FACE('',(#3673),#3128,.T.);
#16790=ADVANCED_FACE('',(#3674),#3129,.T.);
#16791=ADVANCED_FACE('',(#3675),#3130,.T.);
#16792=ADVANCED_FACE('',(#3676),#3131,.T.);
#16793=ADVANCED_FACE('',(#3677),#3132,.T.);
#16794=ADVANCED_FACE('',(#3678),#3133,.T.);
#16795=ADVANCED_FACE('',(#3679),#3134,.T.);
#16796=ADVANCED_FACE('',(#3680),#3135,.T.);
#16797=ADVANCED_FACE('',(#3681),#3136,.T.);
#16798=ADVANCED_FACE('',(#3682),#3137,.T.);
#16799=ADVANCED_FACE('',(#3683),#3138,.T.);
#16800=ADVANCED_FACE('',(#3684),#3139,.T.);
#16801=ADVANCED_FACE('',(#3685),#3140,.T.);
#16802=ADVANCED_FACE('',(#3686),#3141,.T.);
#16803=ADVANCED_FACE('',(#3687),#3142,.T.);
#16804=ADVANCED_FACE('',(#3688),#3143,.T.);
#16805=ADVANCED_FACE('',(#3689),#3144,.T.);
#16806=ADVANCED_FACE('',(#3690),#3145,.T.);
#16807=ADVANCED_FACE('',(#3691),#3146,.T.);
#16808=ADVANCED_FACE('',(#3692),#3147,.T.);
#16809=ADVANCED_FACE('',(#3693),#3148,.T.);
#16810=ADVANCED_FACE('',(#3694),#3149,.T.);
#16811=ADVANCED_FACE('',(#3695),#3150,.T.);
#16812=ADVANCED_FACE('',(#3696),#3151,.T.);
#16813=ADVANCED_FACE('',(#3697),#3152,.T.);
#16814=ADVANCED_FACE('',(#3698),#3153,.T.);
#16815=ADVANCED_FACE('',(#3699),#3154,.T.);
#16816=ADVANCED_FACE('',(#3700),#3155,.T.);
#16817=ADVANCED_FACE('',(#3701),#3156,.T.);
#16818=ADVANCED_FACE('',(#3702),#3157,.T.);
#16819=ADVANCED_FACE('',(#3703),#3158,.T.);
#16820=ADVANCED_FACE('',(#3704),#3159,.T.);
#16821=ADVANCED_FACE('',(#3705),#3160,.T.);
#16822=ADVANCED_FACE('',(#3706),#3161,.T.);
#16823=ADVANCED_FACE('',(#3707),#3162,.T.);
#16824=ADVANCED_FACE('',(#3708),#3163,.T.);
#16825=ADVANCED_FACE('',(#3709),#3164,.T.);
#16826=ADVANCED_FACE('',(#3710),#3165,.T.);
#16827=ADVANCED_FACE('',(#3711),#3166,.T.);
#16828=ADVANCED_FACE('',(#3712),#3167,.T.);
#16829=ADVANCED_FACE('',(#3713),#3168,.T.);
#16830=ADVANCED_FACE('',(#3714),#3169,.T.);
#16831=ADVANCED_FACE('',(#3715),#3170,.T.);
#16832=ADVANCED_FACE('',(#3716),#3171,.T.);
#16833=ADVANCED_FACE('',(#3717),#3172,.T.);
#16834=ADVANCED_FACE('',(#3718),#3173,.T.);
#16835=ADVANCED_FACE('',(#3719),#3174,.T.);
#16836=ADVANCED_FACE('',(#3720),#3175,.T.);
#16837=ADVANCED_FACE('',(#3721),#3176,.T.);
#16838=ADVANCED_FACE('',(#3722),#3177,.T.);
#16839=ADVANCED_FACE('',(#3723),#3178,.T.);
#16840=ADVANCED_FACE('',(#3724),#3179,.T.);
#16841=ADVANCED_FACE('',(#3725),#3180,.T.);
#16842=ADVANCED_FACE('',(#3726),#3181,.T.);
#16843=ADVANCED_FACE('',(#3727),#3182,.T.);
#16844=ADVANCED_FACE('',(#3728),#3183,.T.);
#16845=ADVANCED_FACE('',(#3729),#3184,.T.);
#16846=ADVANCED_FACE('',(#3730),#3185,.F.);
#17666=CLOSED_SHELL('',(#16660,#16661,#16662,#16663,#16664,#16665,#16666,
#16667,#16668,#16669,#16670,#16671,#16672,#16673,#16674,#16675,#16676,#16677,
#16678,#16679,#16680,#16681,#16682,#16683,#16684,#16685,#16686,#16687,#16688,
#16689,#16690,#16691,#16692,#16693,#16694,#16695,#16696,#16697,#16698,#16699,
#16700,#16701,#16702,#16703,#16704,#16705,#16706,#16707,#16708,#16709,#16710,
#16711,#16712,#16713,#16714,#16715,#16716,#16717,#16718,#16719,#16720,#16721,
#16722,#16723,#16724,#16725,#16726,#16727,#16728,#16729,#16730,#16731,#16732,
#16733,#16734,#16735,#16736,#16737,#16738,#16739,#16740,#16741,#16742,#16743,
#16744,#16745,#16746,#16747,#16748,#16749,#16750,#16751,#16752,#16753,#16754,
#16755,#16756,#16757,#16758,#16759,#16760,#16761,#16762,#16763,#16764,#16765,
#16766,#16767,#16768,#16769,#16770,#16771,#16772,#16773,#16774,#16775,#16776,
#16777,#16778,#16779,#16780,#16781,#16782,#16783,#16784,#16785,#16786,#16787,
#16788,#16789,#16790,#16791,#16792,#16793,#16794,#16795,#16796,#16797,#16798,
#16799,#16800,#16801,#16802,#16803,#16804,#16805,#16806,#16807,#16808,#16809,
#16810,#16811,#16812,#16813,#16814,#16815,#16816,#16817,#16818,#16819,#16820,
#16821,#16822,#16823,#16824,#16825,#16826,#16827,#16828,#16829,#16830,#16831,
#16832,#16833,#16834,#16835,#16836,#16837,#16838,#16839,#16840,#16841,#16842,
#16843,#16844,#16845,#16846));
#17836=AXIS2_PLACEMENT_3D('',#23727,#19603,#19604);
#17837=AXIS2_PLACEMENT_3D('',#23728,#19605,#19606);
#17838=AXIS2_PLACEMENT_3D('',#23731,#19607,#19608);
#17839=AXIS2_PLACEMENT_3D('',#23733,#19609,#19610);
#17840=AXIS2_PLACEMENT_3D('',#23735,#19611,#19612);
#17841=AXIS2_PLACEMENT_3D('',#23737,#19613,#19614);
#17842=AXIS2_PLACEMENT_3D('',#23739,#19615,#19616);
#17843=AXIS2_PLACEMENT_3D('',#23741,#19617,#19618);
#17844=AXIS2_PLACEMENT_3D('',#23743,#19619,#19620);
#17845=AXIS2_PLACEMENT_3D('',#23745,#19621,#19622);
#17846=AXIS2_PLACEMENT_3D('',#23747,#19623,#19624);
#17847=AXIS2_PLACEMENT_3D('',#23749,#19625,#19626);
#17848=AXIS2_PLACEMENT_3D('',#23751,#19627,#19628);
#17849=AXIS2_PLACEMENT_3D('',#23753,#19629,#19630);
#17850=AXIS2_PLACEMENT_3D('',#23755,#19631,#19632);
#17851=AXIS2_PLACEMENT_3D('',#23757,#19633,#19634);
#17852=AXIS2_PLACEMENT_3D('',#23759,#19635,#19636);
#17853=AXIS2_PLACEMENT_3D('',#23761,#19637,#19638);
#17854=AXIS2_PLACEMENT_3D('',#23763,#19639,#19640);
#17855=AXIS2_PLACEMENT_3D('',#23765,#19641,#19642);
#17856=AXIS2_PLACEMENT_3D('',#23767,#19643,#19644);
#17857=AXIS2_PLACEMENT_3D('',#23769,#19645,#19646);
#17858=AXIS2_PLACEMENT_3D('',#23771,#19647,#19648);
#17859=AXIS2_PLACEMENT_3D('',#23773,#19649,#19650);
#17860=AXIS2_PLACEMENT_3D('',#23775,#19651,#19652);
#17861=AXIS2_PLACEMENT_3D('',#23777,#19653,#19654);
#17862=AXIS2_PLACEMENT_3D('',#23779,#19655,#19656);
#17863=AXIS2_PLACEMENT_3D('',#23781,#19657,#19658);
#17864=AXIS2_PLACEMENT_3D('',#23783,#19659,#19660);
#17865=AXIS2_PLACEMENT_3D('',#23785,#19661,#19662);
#17866=AXIS2_PLACEMENT_3D('',#23787,#19663,#19664);
#17867=AXIS2_PLACEMENT_3D('',#23789,#19665,#19666);
#17868=AXIS2_PLACEMENT_3D('',#23791,#19667,#19668);
#17869=AXIS2_PLACEMENT_3D('',#23793,#19669,#19670);
#17870=AXIS2_PLACEMENT_3D('',#23795,#19671,#19672);
#17871=AXIS2_PLACEMENT_3D('',#23797,#19673,#19674);
#17872=AXIS2_PLACEMENT_3D('',#23799,#19675,#19676);
#17873=AXIS2_PLACEMENT_3D('',#23801,#19677,#19678);
#17874=AXIS2_PLACEMENT_3D('',#23803,#19679,#19680);
#17875=AXIS2_PLACEMENT_3D('',#23805,#19681,#19682);
#17876=AXIS2_PLACEMENT_3D('',#23807,#19683,#19684);
#17877=AXIS2_PLACEMENT_3D('',#23809,#19685,#19686);
#17878=AXIS2_PLACEMENT_3D('',#23811,#19687,#19688);
#17879=AXIS2_PLACEMENT_3D('',#23813,#19689,#19690);
#17880=AXIS2_PLACEMENT_3D('',#23815,#19691,#19692);
#17881=AXIS2_PLACEMENT_3D('',#23817,#19693,#19694);
#17882=AXIS2_PLACEMENT_3D('',#23819,#19695,#19696);
#17883=AXIS2_PLACEMENT_3D('',#23821,#19697,#19698);
#17884=AXIS2_PLACEMENT_3D('',#23823,#19699,#19700);
#17885=AXIS2_PLACEMENT_3D('',#23825,#19701,#19702);
#17886=AXIS2_PLACEMENT_3D('',#23827,#19703,#19704);
#17887=AXIS2_PLACEMENT_3D('',#23829,#19705,#19706);
#17888=AXIS2_PLACEMENT_3D('',#23831,#19707,#19708);
#17889=AXIS2_PLACEMENT_3D('',#23833,#19709,#19710);
#17890=AXIS2_PLACEMENT_3D('',#23835,#19711,#19712);
#17891=AXIS2_PLACEMENT_3D('',#23837,#19713,#19714);
#17892=AXIS2_PLACEMENT_3D('',#23839,#19715,#19716);
#17893=AXIS2_PLACEMENT_3D('',#23841,#19717,#19718);
#17894=AXIS2_PLACEMENT_3D('',#23843,#19719,#19720);
#17895=AXIS2_PLACEMENT_3D('',#23845,#19721,#19722);
#17896=AXIS2_PLACEMENT_3D('',#23847,#19723,#19724);
#17897=AXIS2_PLACEMENT_3D('',#23849,#19725,#19726);
#17898=AXIS2_PLACEMENT_3D('',#23851,#19727,#19728);
#17899=AXIS2_PLACEMENT_3D('',#23853,#19729,#19730);
#17900=AXIS2_PLACEMENT_3D('',#23855,#19731,#19732);
#17901=AXIS2_PLACEMENT_3D('',#23857,#19733,#19734);
#17902=AXIS2_PLACEMENT_3D('',#23859,#19735,#19736);
#17903=AXIS2_PLACEMENT_3D('',#23861,#19737,#19738);
#17904=AXIS2_PLACEMENT_3D('',#23863,#19739,#19740);
#17905=AXIS2_PLACEMENT_3D('',#23865,#19741,#19742);
#17906=AXIS2_PLACEMENT_3D('',#23867,#19743,#19744);
#17907=AXIS2_PLACEMENT_3D('',#23869,#19745,#19746);
#17908=AXIS2_PLACEMENT_3D('',#23871,#19747,#19748);
#17909=AXIS2_PLACEMENT_3D('',#23873,#19749,#19750);
#17910=AXIS2_PLACEMENT_3D('',#23875,#19751,#19752);
#17911=AXIS2_PLACEMENT_3D('',#23877,#19753,#19754);
#17912=AXIS2_PLACEMENT_3D('',#23879,#19755,#19756);
#17913=AXIS2_PLACEMENT_3D('',#23881,#19757,#19758);
#17914=AXIS2_PLACEMENT_3D('',#23883,#19759,#19760);
#17915=AXIS2_PLACEMENT_3D('',#23885,#19761,#19762);
#17916=AXIS2_PLACEMENT_3D('',#23887,#19763,#19764);
#17917=AXIS2_PLACEMENT_3D('',#23889,#19765,#19766);
#17918=AXIS2_PLACEMENT_3D('',#23891,#19767,#19768);
#17919=AXIS2_PLACEMENT_3D('',#23893,#19769,#19770);
#17920=AXIS2_PLACEMENT_3D('',#23895,#19771,#19772);
#17921=AXIS2_PLACEMENT_3D('',#23897,#19773,#19774);
#17922=AXIS2_PLACEMENT_3D('',#23899,#19775,#19776);
#17923=AXIS2_PLACEMENT_3D('',#23901,#19777,#19778);
#17924=AXIS2_PLACEMENT_3D('',#23903,#19779,#19780);
#17925=AXIS2_PLACEMENT_3D('',#23905,#19781,#19782);
#17926=AXIS2_PLACEMENT_3D('',#23907,#19783,#19784);
#17927=AXIS2_PLACEMENT_3D('',#23909,#19785,#19786);
#17928=AXIS2_PLACEMENT_3D('',#23911,#19787,#19788);
#17929=AXIS2_PLACEMENT_3D('',#23913,#19789,#19790);
#17930=AXIS2_PLACEMENT_3D('',#23915,#19791,#19792);
#17931=AXIS2_PLACEMENT_3D('',#23917,#19793,#19794);
#17932=AXIS2_PLACEMENT_3D('',#23919,#19795,#19796);
#17933=AXIS2_PLACEMENT_3D('',#23921,#19797,#19798);
#17934=AXIS2_PLACEMENT_3D('',#23923,#19799,#19800);
#17935=AXIS2_PLACEMENT_3D('',#23925,#19801,#19802);
#17936=AXIS2_PLACEMENT_3D('',#23927,#19803,#19804);
#17937=AXIS2_PLACEMENT_3D('',#23929,#19805,#19806);
#17938=AXIS2_PLACEMENT_3D('',#23931,#19807,#19808);
#17939=AXIS2_PLACEMENT_3D('',#23933,#19809,#19810);
#17940=AXIS2_PLACEMENT_3D('',#23935,#19811,#19812);
#17941=AXIS2_PLACEMENT_3D('',#23937,#19813,#19814);
#17942=AXIS2_PLACEMENT_3D('',#23939,#19815,#19816);
#17943=AXIS2_PLACEMENT_3D('',#23941,#19817,#19818);
#17944=AXIS2_PLACEMENT_3D('',#23943,#19819,#19820);
#17945=AXIS2_PLACEMENT_3D('',#23945,#19821,#19822);
#17946=AXIS2_PLACEMENT_3D('',#23947,#19823,#19824);
#17947=AXIS2_PLACEMENT_3D('',#23949,#19825,#19826);
#17948=AXIS2_PLACEMENT_3D('',#23951,#19827,#19828);
#17949=AXIS2_PLACEMENT_3D('',#23953,#19829,#19830);
#17950=AXIS2_PLACEMENT_3D('',#23955,#19831,#19832);
#17951=AXIS2_PLACEMENT_3D('',#23957,#19833,#19834);
#17952=AXIS2_PLACEMENT_3D('',#23959,#19835,#19836);
#17953=AXIS2_PLACEMENT_3D('',#23961,#19837,#19838);
#17954=AXIS2_PLACEMENT_3D('',#23963,#19839,#19840);
#17955=AXIS2_PLACEMENT_3D('',#23965,#19841,#19842);
#17956=AXIS2_PLACEMENT_3D('',#23967,#19843,#19844);
#17957=AXIS2_PLACEMENT_3D('',#23969,#19845,#19846);
#17958=AXIS2_PLACEMENT_3D('',#23971,#19847,#19848);
#17959=AXIS2_PLACEMENT_3D('',#23973,#19849,#19850);
#17960=AXIS2_PLACEMENT_3D('',#23975,#19851,#19852);
#17961=AXIS2_PLACEMENT_3D('',#23977,#19853,#19854);
#17962=AXIS2_PLACEMENT_3D('',#23979,#19855,#19856);
#17963=AXIS2_PLACEMENT_3D('',#23981,#19857,#19858);
#17964=AXIS2_PLACEMENT_3D('',#23983,#19859,#19860);
#17965=AXIS2_PLACEMENT_3D('',#23985,#19861,#19862);
#17966=AXIS2_PLACEMENT_3D('',#23987,#19863,#19864);
#17967=AXIS2_PLACEMENT_3D('',#23989,#19865,#19866);
#17968=AXIS2_PLACEMENT_3D('',#23991,#19867,#19868);
#17969=AXIS2_PLACEMENT_3D('',#23993,#19869,#19870);
#17970=AXIS2_PLACEMENT_3D('',#23995,#19871,#19872);
#17971=AXIS2_PLACEMENT_3D('',#23997,#19873,#19874);
#17972=AXIS2_PLACEMENT_3D('',#23999,#19875,#19876);
#17973=AXIS2_PLACEMENT_3D('',#24001,#19877,#19878);
#17974=AXIS2_PLACEMENT_3D('',#24003,#19879,#19880);
#17975=AXIS2_PLACEMENT_3D('',#24005,#19881,#19882);
#17976=AXIS2_PLACEMENT_3D('',#24007,#19883,#19884);
#17977=AXIS2_PLACEMENT_3D('',#24009,#19885,#19886);
#17978=AXIS2_PLACEMENT_3D('',#24011,#19887,#19888);
#17979=AXIS2_PLACEMENT_3D('',#24013,#19889,#19890);
#17980=AXIS2_PLACEMENT_3D('',#24015,#19891,#19892);
#17981=AXIS2_PLACEMENT_3D('',#24017,#19893,#19894);
#17982=AXIS2_PLACEMENT_3D('',#24019,#19895,#19896);
#17983=AXIS2_PLACEMENT_3D('',#24021,#19897,#19898);
#17984=AXIS2_PLACEMENT_3D('',#24023,#19899,#19900);
#17985=AXIS2_PLACEMENT_3D('',#24025,#19901,#19902);
#17986=AXIS2_PLACEMENT_3D('',#24027,#19903,#19904);
#17987=AXIS2_PLACEMENT_3D('',#24029,#19905,#19906);
#17988=AXIS2_PLACEMENT_3D('',#24031,#19907,#19908);
#17989=AXIS2_PLACEMENT_3D('',#24033,#19909,#19910);
#17990=AXIS2_PLACEMENT_3D('',#24035,#19911,#19912);
#17991=AXIS2_PLACEMENT_3D('',#24037,#19913,#19914);
#17992=AXIS2_PLACEMENT_3D('',#24039,#19915,#19916);
#17993=AXIS2_PLACEMENT_3D('',#24041,#19917,#19918);
#17994=AXIS2_PLACEMENT_3D('',#24043,#19919,#19920);
#17995=AXIS2_PLACEMENT_3D('',#24045,#19921,#19922);
#17996=AXIS2_PLACEMENT_3D('',#24047,#19923,#19924);
#17997=AXIS2_PLACEMENT_3D('',#24049,#19925,#19926);
#17998=AXIS2_PLACEMENT_3D('',#24051,#19927,#19928);
#17999=AXIS2_PLACEMENT_3D('',#24053,#19929,#19930);
#18000=AXIS2_PLACEMENT_3D('',#24055,#19931,#19932);
#18001=AXIS2_PLACEMENT_3D('',#24057,#19933,#19934);
#18002=AXIS2_PLACEMENT_3D('',#24059,#19935,#19936);
#18003=AXIS2_PLACEMENT_3D('',#24061,#19937,#19938);
#18004=AXIS2_PLACEMENT_3D('',#24063,#19939,#19940);
#18005=AXIS2_PLACEMENT_3D('',#24065,#19941,#19942);
#18006=AXIS2_PLACEMENT_3D('',#24067,#19943,#19944);
#18007=AXIS2_PLACEMENT_3D('',#24069,#19945,#19946);
#18008=AXIS2_PLACEMENT_3D('',#24071,#19947,#19948);
#18009=AXIS2_PLACEMENT_3D('',#24073,#19949,#19950);
#18010=AXIS2_PLACEMENT_3D('',#24075,#19951,#19952);
#18011=AXIS2_PLACEMENT_3D('',#24077,#19953,#19954);
#18012=AXIS2_PLACEMENT_3D('',#24079,#19955,#19956);
#18013=AXIS2_PLACEMENT_3D('',#24081,#19957,#19958);
#18014=AXIS2_PLACEMENT_3D('',#24083,#19959,#19960);
#18015=AXIS2_PLACEMENT_3D('',#24085,#19961,#19962);
#18016=AXIS2_PLACEMENT_3D('',#24087,#19963,#19964);
#18017=AXIS2_PLACEMENT_3D('',#24089,#19965,#19966);
#18018=AXIS2_PLACEMENT_3D('',#24091,#19967,#19968);
#18019=AXIS2_PLACEMENT_3D('',#24093,#19969,#19970);
#18020=AXIS2_PLACEMENT_3D('',#24095,#19971,#19972);
#18021=AXIS2_PLACEMENT_3D('',#24096,#19973,#19974);
#18022=AXIS2_PLACEMENT_3D('',#24098,#19975,#19976);
#18023=AXIS2_PLACEMENT_3D('',#24099,#19977,#19978);
#18024=AXIS2_PLACEMENT_3D('',#24104,#19981,#19982);
#18025=AXIS2_PLACEMENT_3D('',#24105,#19983,#19984);
#18026=AXIS2_PLACEMENT_3D('',#24109,#19986,#19987);
#18027=AXIS2_PLACEMENT_3D('',#24111,#19989,#19990);
#18028=AXIS2_PLACEMENT_3D('',#24116,#19993,#19994);
#18029=AXIS2_PLACEMENT_3D('',#24117,#19995,#19996);
#18030=AXIS2_PLACEMENT_3D('',#24122,#19999,#20000);
#18031=AXIS2_PLACEMENT_3D('',#24123,#20001,#20002);
#18032=AXIS2_PLACEMENT_3D('',#24128,#20005,#20006);
#18033=AXIS2_PLACEMENT_3D('',#24129,#20007,#20008);
#18034=AXIS2_PLACEMENT_3D('',#24133,#20010,#20011);
#18035=AXIS2_PLACEMENT_3D('',#24135,#20013,#20014);
#18036=AXIS2_PLACEMENT_3D('',#24139,#20016,#20017);
#18037=AXIS2_PLACEMENT_3D('',#24141,#20019,#20020);
#18038=AXIS2_PLACEMENT_3D('',#24146,#20023,#20024);
#18039=AXIS2_PLACEMENT_3D('',#24147,#20025,#20026);
#18040=AXIS2_PLACEMENT_3D('',#24151,#20028,#20029);
#18041=AXIS2_PLACEMENT_3D('',#24153,#20031,#20032);
#18042=AXIS2_PLACEMENT_3D('',#24158,#20035,#20036);
#18043=AXIS2_PLACEMENT_3D('',#24159,#20037,#20038);
#18044=AXIS2_PLACEMENT_3D('',#24164,#20041,#20042);
#18045=AXIS2_PLACEMENT_3D('',#24165,#20043,#20044);
#18046=AXIS2_PLACEMENT_3D('',#24170,#20047,#20048);
#18047=AXIS2_PLACEMENT_3D('',#24171,#20049,#20050);
#18048=AXIS2_PLACEMENT_3D('',#24176,#20053,#20054);
#18049=AXIS2_PLACEMENT_3D('',#24177,#20055,#20056);
#18050=AXIS2_PLACEMENT_3D('',#24181,#20058,#20059);
#18051=AXIS2_PLACEMENT_3D('',#24183,#20061,#20062);
#18052=AXIS2_PLACEMENT_3D('',#24188,#20065,#20066);
#18053=AXIS2_PLACEMENT_3D('',#24189,#20067,#20068);
#18054=AXIS2_PLACEMENT_3D('',#24194,#20071,#20072);
#18055=AXIS2_PLACEMENT_3D('',#24195,#20073,#20074);
#18056=AXIS2_PLACEMENT_3D('',#24200,#20077,#20078);
#18057=AXIS2_PLACEMENT_3D('',#24201,#20079,#20080);
#18058=AXIS2_PLACEMENT_3D('',#24205,#20082,#20083);
#18059=AXIS2_PLACEMENT_3D('',#24207,#20085,#20086);
#18060=AXIS2_PLACEMENT_3D('',#24211,#20088,#20089);
#18061=AXIS2_PLACEMENT_3D('',#24213,#20091,#20092);
#18062=AXIS2_PLACEMENT_3D('',#24218,#20095,#20096);
#18063=AXIS2_PLACEMENT_3D('',#24219,#20097,#20098);
#18064=AXIS2_PLACEMENT_3D('',#24223,#20100,#20101);
#18065=AXIS2_PLACEMENT_3D('',#24225,#20103,#20104);
#18066=AXIS2_PLACEMENT_3D('',#24230,#20107,#20108);
#18067=AXIS2_PLACEMENT_3D('',#24231,#20109,#20110);
#18068=AXIS2_PLACEMENT_3D('',#24236,#20113,#20114);
#18069=AXIS2_PLACEMENT_3D('',#24237,#20115,#20116);
#18070=AXIS2_PLACEMENT_3D('',#24242,#20119,#20120);
#18071=AXIS2_PLACEMENT_3D('',#24243,#20121,#20122);
#18072=AXIS2_PLACEMENT_3D('',#24247,#20124,#20125);
#18073=AXIS2_PLACEMENT_3D('',#24249,#20127,#20128);
#18074=AXIS2_PLACEMENT_3D('',#24254,#20131,#20132);
#18075=AXIS2_PLACEMENT_3D('',#24255,#20133,#20134);
#18076=AXIS2_PLACEMENT_3D('',#24260,#20137,#20138);
#18077=AXIS2_PLACEMENT_3D('',#24261,#20139,#20140);
#18078=AXIS2_PLACEMENT_3D('',#24266,#20143,#20144);
#18079=AXIS2_PLACEMENT_3D('',#24267,#20145,#20146);
#18080=AXIS2_PLACEMENT_3D('',#24271,#20148,#20149);
#18081=AXIS2_PLACEMENT_3D('',#24273,#20151,#20152);
#18082=AXIS2_PLACEMENT_3D('',#24278,#20155,#20156);
#18083=AXIS2_PLACEMENT_3D('',#24279,#20157,#20158);
#18084=AXIS2_PLACEMENT_3D('',#24284,#20161,#20162);
#18085=AXIS2_PLACEMENT_3D('',#24285,#20163,#20164);
#18086=AXIS2_PLACEMENT_3D('',#24289,#20166,#20167);
#18087=AXIS2_PLACEMENT_3D('',#24291,#20169,#20170);
#18088=AXIS2_PLACEMENT_3D('',#24296,#20173,#20174);
#18089=AXIS2_PLACEMENT_3D('',#24297,#20175,#20176);
#18090=AXIS2_PLACEMENT_3D('',#24302,#20179,#20180);
#18091=AXIS2_PLACEMENT_3D('',#24303,#20181,#20182);
#18092=AXIS2_PLACEMENT_3D('',#24308,#20185,#20186);
#18093=AXIS2_PLACEMENT_3D('',#24309,#20187,#20188);
#18094=AXIS2_PLACEMENT_3D('',#24313,#20190,#20191);
#18095=AXIS2_PLACEMENT_3D('',#24315,#20193,#20194);
#18096=AXIS2_PLACEMENT_3D('',#24320,#20197,#20198);
#18097=AXIS2_PLACEMENT_3D('',#24321,#20199,#20200);
#18098=AXIS2_PLACEMENT_3D('',#24326,#20203,#20204);
#18099=AXIS2_PLACEMENT_3D('',#24327,#20205,#20206);
#18100=AXIS2_PLACEMENT_3D('',#24332,#20209,#20210);
#18101=AXIS2_PLACEMENT_3D('',#24333,#20211,#20212);
#18102=AXIS2_PLACEMENT_3D('',#24337,#20214,#20215);
#18103=AXIS2_PLACEMENT_3D('',#24339,#20217,#20218);
#18104=AXIS2_PLACEMENT_3D('',#24344,#20221,#20222);
#18105=AXIS2_PLACEMENT_3D('',#24345,#20223,#20224);
#18106=AXIS2_PLACEMENT_3D('',#24350,#20227,#20228);
#18107=AXIS2_PLACEMENT_3D('',#24351,#20229,#20230);
#18108=AXIS2_PLACEMENT_3D('',#24355,#20232,#20233);
#18109=AXIS2_PLACEMENT_3D('',#24357,#20235,#20236);
#18110=AXIS2_PLACEMENT_3D('',#24362,#20239,#20240);
#18111=AXIS2_PLACEMENT_3D('',#24363,#20241,#20242);
#18112=AXIS2_PLACEMENT_3D('',#24368,#20245,#20246);
#18113=AXIS2_PLACEMENT_3D('',#24369,#20247,#20248);
#18114=AXIS2_PLACEMENT_3D('',#24371,#20249,#20250);
#18115=AXIS2_PLACEMENT_3D('',#24373,#20251,#20252);
#18116=AXIS2_PLACEMENT_3D('',#24375,#20253,#20254);
#18117=AXIS2_PLACEMENT_3D('',#24376,#20255,#20256);
#18118=AXIS2_PLACEMENT_3D('',#24378,#20257,#20258);
#18119=AXIS2_PLACEMENT_3D('',#24380,#20259,#20260);
#18120=AXIS2_PLACEMENT_3D('',#24381,#20261,#20262);
#18121=AXIS2_PLACEMENT_3D('',#24383,#20263,#20264);
#18122=AXIS2_PLACEMENT_3D('',#24385,#20265,#20266);
#18123=AXIS2_PLACEMENT_3D('',#24386,#20267,#20268);
#18124=AXIS2_PLACEMENT_3D('',#24388,#20269,#20270);
#18125=AXIS2_PLACEMENT_3D('',#24390,#20271,#20272);
#18126=AXIS2_PLACEMENT_3D('',#24391,#20273,#20274);
#18127=AXIS2_PLACEMENT_3D('',#24393,#20275,#20276);
#18128=AXIS2_PLACEMENT_3D('',#24395,#20277,#20278);
#18129=AXIS2_PLACEMENT_3D('',#24396,#20279,#20280);
#18130=AXIS2_PLACEMENT_3D('',#24398,#20281,#20282);
#18131=AXIS2_PLACEMENT_3D('',#24400,#20283,#20284);
#18132=AXIS2_PLACEMENT_3D('',#24401,#20285,#20286);
#18133=AXIS2_PLACEMENT_3D('',#24403,#20287,#20288);
#18134=AXIS2_PLACEMENT_3D('',#24405,#20289,#20290);
#18135=AXIS2_PLACEMENT_3D('',#24406,#20291,#20292);
#18136=AXIS2_PLACEMENT_3D('',#24408,#20293,#20294);
#18137=AXIS2_PLACEMENT_3D('',#24410,#20295,#20296);
#18138=AXIS2_PLACEMENT_3D('',#24411,#20297,#20298);
#18139=AXIS2_PLACEMENT_3D('',#24413,#20299,#20300);
#18140=AXIS2_PLACEMENT_3D('',#24415,#20301,#20302);
#18141=AXIS2_PLACEMENT_3D('',#24416,#20303,#20304);
#18142=AXIS2_PLACEMENT_3D('',#24418,#20305,#20306);
#18143=AXIS2_PLACEMENT_3D('',#24420,#20307,#20308);
#18144=AXIS2_PLACEMENT_3D('',#24421,#20309,#20310);
#18145=AXIS2_PLACEMENT_3D('',#24423,#20311,#20312);
#18146=AXIS2_PLACEMENT_3D('',#24425,#20313,#20314);
#18147=AXIS2_PLACEMENT_3D('',#24427,#20315,#20316);
#18148=AXIS2_PLACEMENT_3D('',#24429,#20317,#20318);
#18149=AXIS2_PLACEMENT_3D('',#24431,#20319,#20320);
#18150=AXIS2_PLACEMENT_3D('',#24433,#20321,#20322);
#18151=AXIS2_PLACEMENT_3D('',#24434,#20323,#20324);
#18152=AXIS2_PLACEMENT_3D('',#24436,#20325,#20326);
#18153=AXIS2_PLACEMENT_3D('',#24438,#20327,#20328);
#18154=AXIS2_PLACEMENT_3D('',#24439,#20329,#20330);
#18155=AXIS2_PLACEMENT_3D('',#24441,#20331,#20332);
#18156=AXIS2_PLACEMENT_3D('',#24443,#20333,#20334);
#18157=AXIS2_PLACEMENT_3D('',#24444,#20335,#20336);
#18158=AXIS2_PLACEMENT_3D('',#24446,#20337,#20338);
#18159=AXIS2_PLACEMENT_3D('',#24448,#20339,#20340);
#18160=AXIS2_PLACEMENT_3D('',#24449,#20341,#20342);
#18161=AXIS2_PLACEMENT_3D('',#24451,#20343,#20344);
#18162=AXIS2_PLACEMENT_3D('',#24453,#20345,#20346);
#18163=AXIS2_PLACEMENT_3D('',#24454,#20347,#20348);
#18164=AXIS2_PLACEMENT_3D('',#24456,#20349,#20350);
#18165=AXIS2_PLACEMENT_3D('',#24458,#20351,#20352);
#18166=AXIS2_PLACEMENT_3D('',#24459,#20353,#20354);
#18167=AXIS2_PLACEMENT_3D('',#24461,#20355,#20356);
#18168=AXIS2_PLACEMENT_3D('',#24463,#20357,#20358);
#18169=AXIS2_PLACEMENT_3D('',#24464,#20359,#20360);
#18170=AXIS2_PLACEMENT_3D('',#24466,#20361,#20362);
#18171=AXIS2_PLACEMENT_3D('',#24468,#20363,#20364);
#18172=AXIS2_PLACEMENT_3D('',#24469,#20365,#20366);
#18173=AXIS2_PLACEMENT_3D('',#24471,#20367,#20368);
#18174=AXIS2_PLACEMENT_3D('',#24473,#20369,#20370);
#18175=AXIS2_PLACEMENT_3D('',#24474,#20371,#20372);
#18176=AXIS2_PLACEMENT_3D('',#24476,#20373,#20374);
#18177=AXIS2_PLACEMENT_3D('',#24478,#20375,#20376);
#18178=AXIS2_PLACEMENT_3D('',#24479,#20377,#20378);
#18179=AXIS2_PLACEMENT_3D('',#24481,#20379,#20380);
#18180=AXIS2_PLACEMENT_3D('',#24483,#20381,#20382);
#18181=AXIS2_PLACEMENT_3D('',#24484,#20383,#20384);
#18182=AXIS2_PLACEMENT_3D('',#24486,#20385,#20386);
#18183=AXIS2_PLACEMENT_3D('',#24488,#20387,#20388);
#18184=AXIS2_PLACEMENT_3D('',#24489,#20389,#20390);
#18185=AXIS2_PLACEMENT_3D('',#24491,#20391,#20392);
#18186=AXIS2_PLACEMENT_3D('',#24493,#20393,#20394);
#18187=AXIS2_PLACEMENT_3D('',#24494,#20395,#20396);
#18188=AXIS2_PLACEMENT_3D('',#24496,#20397,#20398);
#18189=AXIS2_PLACEMENT_3D('',#24498,#20399,#20400);
#18190=AXIS2_PLACEMENT_3D('',#24499,#20401,#20402);
#18191=AXIS2_PLACEMENT_3D('',#24501,#20403,#20404);
#18192=AXIS2_PLACEMENT_3D('',#24503,#20405,#20406);
#18193=AXIS2_PLACEMENT_3D('',#24504,#20407,#20408);
#18194=AXIS2_PLACEMENT_3D('',#24506,#20409,#20410);
#18195=AXIS2_PLACEMENT_3D('',#24508,#20411,#20412);
#18196=AXIS2_PLACEMENT_3D('',#24509,#20413,#20414);
#18197=AXIS2_PLACEMENT_3D('',#24511,#20415,#20416);
#18198=AXIS2_PLACEMENT_3D('',#24513,#20417,#20418);
#18199=AXIS2_PLACEMENT_3D('',#24514,#20419,#20420);
#18200=AXIS2_PLACEMENT_3D('',#24516,#20421,#20422);
#18201=AXIS2_PLACEMENT_3D('',#24518,#20423,#20424);
#18202=AXIS2_PLACEMENT_3D('',#24519,#20425,#20426);
#18203=AXIS2_PLACEMENT_3D('',#24521,#20427,#20428);
#18204=AXIS2_PLACEMENT_3D('',#24523,#20429,#20430);
#18205=AXIS2_PLACEMENT_3D('',#24524,#20431,#20432);
#18206=AXIS2_PLACEMENT_3D('',#24526,#20433,#20434);
#18207=AXIS2_PLACEMENT_3D('',#24528,#20435,#20436);
#18208=AXIS2_PLACEMENT_3D('',#24529,#20437,#20438);
#18209=AXIS2_PLACEMENT_3D('',#24531,#20439,#20440);
#18210=AXIS2_PLACEMENT_3D('',#24533,#20441,#20442);
#18211=AXIS2_PLACEMENT_3D('',#24534,#20443,#20444);
#18212=AXIS2_PLACEMENT_3D('',#24536,#20445,#20446);
#18213=AXIS2_PLACEMENT_3D('',#24538,#20447,#20448);
#18214=AXIS2_PLACEMENT_3D('',#24539,#20449,#20450);
#18215=AXIS2_PLACEMENT_3D('',#24541,#20451,#20452);
#18216=AXIS2_PLACEMENT_3D('',#24543,#20453,#20454);
#18217=AXIS2_PLACEMENT_3D('',#24544,#20455,#20456);
#18218=AXIS2_PLACEMENT_3D('',#24546,#20457,#20458);
#18219=AXIS2_PLACEMENT_3D('',#24548,#20459,#20460);
#18220=AXIS2_PLACEMENT_3D('',#24549,#20461,#20462);
#18221=AXIS2_PLACEMENT_3D('',#24551,#20463,#20464);
#18222=AXIS2_PLACEMENT_3D('',#24553,#20465,#20466);
#18223=AXIS2_PLACEMENT_3D('',#24554,#20467,#20468);
#18224=AXIS2_PLACEMENT_3D('',#24556,#20469,#20470);
#18225=AXIS2_PLACEMENT_3D('',#24558,#20471,#20472);
#18226=AXIS2_PLACEMENT_3D('',#24559,#20473,#20474);
#18227=AXIS2_PLACEMENT_3D('',#24561,#20475,#20476);
#18228=AXIS2_PLACEMENT_3D('',#24563,#20477,#20478);
#18229=AXIS2_PLACEMENT_3D('',#24564,#20479,#20480);
#18230=AXIS2_PLACEMENT_3D('',#24566,#20481,#20482);
#18231=AXIS2_PLACEMENT_3D('',#24568,#20483,#20484);
#18232=AXIS2_PLACEMENT_3D('',#24569,#20485,#20486);
#18233=AXIS2_PLACEMENT_3D('',#24571,#20487,#20488);
#18234=AXIS2_PLACEMENT_3D('',#24573,#20489,#20490);
#18235=AXIS2_PLACEMENT_3D('',#24574,#20491,#20492);
#18236=AXIS2_PLACEMENT_3D('',#24576,#20493,#20494);
#18237=AXIS2_PLACEMENT_3D('',#24578,#20495,#20496);
#18238=AXIS2_PLACEMENT_3D('',#24579,#20497,#20498);
#18239=AXIS2_PLACEMENT_3D('',#24581,#20499,#20500);
#18240=AXIS2_PLACEMENT_3D('',#24583,#20501,#20502);
#18241=AXIS2_PLACEMENT_3D('',#24584,#20503,#20504);
#18242=AXIS2_PLACEMENT_3D('',#24586,#20505,#20506);
#18243=AXIS2_PLACEMENT_3D('',#24588,#20507,#20508);
#18244=AXIS2_PLACEMENT_3D('',#24589,#20509,#20510);
#18245=AXIS2_PLACEMENT_3D('',#24591,#20511,#20512);
#18246=AXIS2_PLACEMENT_3D('',#24593,#20513,#20514);
#18247=AXIS2_PLACEMENT_3D('',#24594,#20515,#20516);
#18248=AXIS2_PLACEMENT_3D('',#24596,#20517,#20518);
#18249=AXIS2_PLACEMENT_3D('',#24598,#20519,#20520);
#18250=AXIS2_PLACEMENT_3D('',#24599,#20521,#20522);
#18251=AXIS2_PLACEMENT_3D('',#24601,#20523,#20524);
#18252=AXIS2_PLACEMENT_3D('',#24602,#20525,#20526);
#18253=AXIS2_PLACEMENT_3D('',#24604,#20527,#20528);
#18254=AXIS2_PLACEMENT_3D('',#24605,#20529,#20530);
#18255=AXIS2_PLACEMENT_3D('',#24608,#20533,#20534);
#18256=AXIS2_PLACEMENT_3D('',#24610,#20536,#20537);
#18257=AXIS2_PLACEMENT_3D('',#24612,#20539,#20540);
#18258=AXIS2_PLACEMENT_3D('',#24613,#20541,#20542);
#18259=AXIS2_PLACEMENT_3D('',#24615,#20544,#20545);
#18260=AXIS2_PLACEMENT_3D('',#24617,#20547,#20548);
#18261=AXIS2_PLACEMENT_3D('',#24618,#20549,#20550);
#18262=AXIS2_PLACEMENT_3D('',#24620,#20552,#20553);
#18263=AXIS2_PLACEMENT_3D('',#24622,#20555,#20556);
#18264=AXIS2_PLACEMENT_3D('',#24623,#20557,#20558);
#18265=AXIS2_PLACEMENT_3D('',#24625,#20560,#20561);
#18266=AXIS2_PLACEMENT_3D('',#24627,#20563,#20564);
#18267=AXIS2_PLACEMENT_3D('',#24628,#20565,#20566);
#18268=AXIS2_PLACEMENT_3D('',#24630,#20568,#20569);
#18269=AXIS2_PLACEMENT_3D('',#24632,#20571,#20572);
#18270=AXIS2_PLACEMENT_3D('',#24633,#20573,#20574);
#18271=AXIS2_PLACEMENT_3D('',#24635,#20576,#20577);
#18272=AXIS2_PLACEMENT_3D('',#24637,#20579,#20580);
#18273=AXIS2_PLACEMENT_3D('',#24638,#20581,#20582);
#18274=AXIS2_PLACEMENT_3D('',#24640,#20584,#20585);
#18275=AXIS2_PLACEMENT_3D('',#24642,#20587,#20588);
#18276=AXIS2_PLACEMENT_3D('',#24643,#20589,#20590);
#18277=AXIS2_PLACEMENT_3D('',#24645,#20592,#20593);
#18278=AXIS2_PLACEMENT_3D('',#24647,#20595,#20596);
#18279=AXIS2_PLACEMENT_3D('',#24648,#20597,#20598);
#18280=AXIS2_PLACEMENT_3D('',#24650,#20600,#20601);
#18281=AXIS2_PLACEMENT_3D('',#24652,#20603,#20604);
#18282=AXIS2_PLACEMENT_3D('',#24653,#20605,#20606);
#18283=AXIS2_PLACEMENT_3D('',#24655,#20608,#20609);
#18284=AXIS2_PLACEMENT_3D('',#24657,#20611,#20612);
#18285=AXIS2_PLACEMENT_3D('',#24658,#20613,#20614);
#18286=AXIS2_PLACEMENT_3D('',#24660,#20616,#20617);
#18287=AXIS2_PLACEMENT_3D('',#24662,#20619,#20620);
#18288=AXIS2_PLACEMENT_3D('',#24663,#20621,#20622);
#18289=AXIS2_PLACEMENT_3D('',#24665,#20624,#20625);
#18290=AXIS2_PLACEMENT_3D('',#24667,#20627,#20628);
#18291=AXIS2_PLACEMENT_3D('',#24668,#20629,#20630);
#18292=AXIS2_PLACEMENT_3D('',#24670,#20632,#20633);
#18293=AXIS2_PLACEMENT_3D('',#24672,#20635,#20636);
#18294=AXIS2_PLACEMENT_3D('',#24673,#20637,#20638);
#18295=AXIS2_PLACEMENT_3D('',#24675,#20640,#20641);
#18296=AXIS2_PLACEMENT_3D('',#24677,#20643,#20644);
#18297=AXIS2_PLACEMENT_3D('',#24678,#20645,#20646);
#18298=AXIS2_PLACEMENT_3D('',#24680,#20648,#20649);
#18299=AXIS2_PLACEMENT_3D('',#24682,#20651,#20652);
#18300=AXIS2_PLACEMENT_3D('',#24683,#20653,#20654);
#18301=AXIS2_PLACEMENT_3D('',#24685,#20656,#20657);
#18302=AXIS2_PLACEMENT_3D('',#24687,#20659,#20660);
#18303=AXIS2_PLACEMENT_3D('',#24688,#20661,#20662);
#18304=AXIS2_PLACEMENT_3D('',#24690,#20664,#20665);
#18305=AXIS2_PLACEMENT_3D('',#24692,#20667,#20668);
#18306=AXIS2_PLACEMENT_3D('',#24693,#20669,#20670);
#18307=AXIS2_PLACEMENT_3D('',#24695,#20672,#20673);
#18308=AXIS2_PLACEMENT_3D('',#24697,#20675,#20676);
#18309=AXIS2_PLACEMENT_3D('',#24698,#20677,#20678);
#18310=AXIS2_PLACEMENT_3D('',#24700,#20680,#20681);
#18311=AXIS2_PLACEMENT_3D('',#24702,#20683,#20684);
#18312=AXIS2_PLACEMENT_3D('',#24703,#20685,#20686);
#18313=AXIS2_PLACEMENT_3D('',#24705,#20688,#20689);
#18314=AXIS2_PLACEMENT_3D('',#24707,#20691,#20692);
#18315=AXIS2_PLACEMENT_3D('',#24708,#20693,#20694);
#18316=AXIS2_PLACEMENT_3D('',#24710,#20696,#20697);
#18317=AXIS2_PLACEMENT_3D('',#24712,#20699,#20700);
#18318=AXIS2_PLACEMENT_3D('',#24713,#20701,#20702);
#18319=AXIS2_PLACEMENT_3D('',#24715,#20704,#20705);
#18320=AXIS2_PLACEMENT_3D('',#24717,#20707,#20708);
#18321=AXIS2_PLACEMENT_3D('',#24718,#20709,#20710);
#18322=AXIS2_PLACEMENT_3D('',#24720,#20712,#20713);
#18323=AXIS2_PLACEMENT_3D('',#24722,#20715,#20716);
#18324=AXIS2_PLACEMENT_3D('',#24723,#20717,#20718);
#18325=AXIS2_PLACEMENT_3D('',#24725,#20720,#20721);
#18326=AXIS2_PLACEMENT_3D('',#24727,#20723,#20724);
#18327=AXIS2_PLACEMENT_3D('',#24728,#20725,#20726);
#18328=AXIS2_PLACEMENT_3D('',#24730,#20728,#20729);
#18329=AXIS2_PLACEMENT_3D('',#24732,#20731,#20732);
#18330=AXIS2_PLACEMENT_3D('',#24733,#20733,#20734);
#18331=AXIS2_PLACEMENT_3D('',#24735,#20736,#20737);
#18332=AXIS2_PLACEMENT_3D('',#24737,#20739,#20740);
#18333=AXIS2_PLACEMENT_3D('',#24738,#20741,#20742);
#18334=AXIS2_PLACEMENT_3D('',#24740,#20744,#20745);
#18335=AXIS2_PLACEMENT_3D('',#24742,#20747,#20748);
#18336=AXIS2_PLACEMENT_3D('',#24743,#20749,#20750);
#18337=AXIS2_PLACEMENT_3D('',#24745,#20752,#20753);
#18338=AXIS2_PLACEMENT_3D('',#24747,#20755,#20756);
#18339=AXIS2_PLACEMENT_3D('',#24748,#20757,#20758);
#18340=AXIS2_PLACEMENT_3D('',#24750,#20760,#20761);
#18341=AXIS2_PLACEMENT_3D('',#24752,#20763,#20764);
#18342=AXIS2_PLACEMENT_3D('',#24753,#20765,#20766);
#18343=AXIS2_PLACEMENT_3D('',#24755,#20768,#20769);
#18344=AXIS2_PLACEMENT_3D('',#24757,#20771,#20772);
#18345=AXIS2_PLACEMENT_3D('',#24758,#20773,#20774);
#18346=AXIS2_PLACEMENT_3D('',#24760,#20776,#20777);
#18347=AXIS2_PLACEMENT_3D('',#24762,#20779,#20780);
#18348=AXIS2_PLACEMENT_3D('',#24763,#20781,#20782);
#18349=AXIS2_PLACEMENT_3D('',#24765,#20784,#20785);
#18350=AXIS2_PLACEMENT_3D('',#24767,#20787,#20788);
#18351=AXIS2_PLACEMENT_3D('',#24768,#20789,#20790);
#18352=AXIS2_PLACEMENT_3D('',#24770,#20792,#20793);
#18353=AXIS2_PLACEMENT_3D('',#24772,#20795,#20796);
#18354=AXIS2_PLACEMENT_3D('',#24773,#20797,#20798);
#18355=AXIS2_PLACEMENT_3D('',#24775,#20800,#20801);
#18356=AXIS2_PLACEMENT_3D('',#24777,#20803,#20804);
#18357=AXIS2_PLACEMENT_3D('',#24778,#20805,#20806);
#18358=AXIS2_PLACEMENT_3D('',#24780,#20808,#20809);
#18359=AXIS2_PLACEMENT_3D('',#24782,#20811,#20812);
#18360=AXIS2_PLACEMENT_3D('',#24783,#20813,#20814);
#18361=AXIS2_PLACEMENT_3D('',#24785,#20816,#20817);
#18362=AXIS2_PLACEMENT_3D('',#24787,#20819,#20820);
#18363=AXIS2_PLACEMENT_3D('',#24788,#20821,#20822);
#18364=AXIS2_PLACEMENT_3D('',#24790,#20824,#20825);
#18365=AXIS2_PLACEMENT_3D('',#24792,#20827,#20828);
#18366=AXIS2_PLACEMENT_3D('',#24793,#20829,#20830);
#18367=AXIS2_PLACEMENT_3D('',#24795,#20832,#20833);
#18368=AXIS2_PLACEMENT_3D('',#24797,#20835,#20836);
#18369=AXIS2_PLACEMENT_3D('',#24798,#20837,#20838);
#18370=AXIS2_PLACEMENT_3D('',#24800,#20840,#20841);
#18371=AXIS2_PLACEMENT_3D('',#24802,#20843,#20844);
#18372=AXIS2_PLACEMENT_3D('',#24803,#20845,#20846);
#18373=AXIS2_PLACEMENT_3D('',#24805,#20848,#20849);
#18374=AXIS2_PLACEMENT_3D('',#24807,#20851,#20852);
#18375=AXIS2_PLACEMENT_3D('',#24808,#20853,#20854);
#18376=AXIS2_PLACEMENT_3D('',#24810,#20856,#20857);
#18377=AXIS2_PLACEMENT_3D('',#24812,#20859,#20860);
#18378=AXIS2_PLACEMENT_3D('',#24813,#20861,#20862);
#18379=AXIS2_PLACEMENT_3D('',#24815,#20864,#20865);
#18380=AXIS2_PLACEMENT_3D('',#24817,#20867,#20868);
#18381=AXIS2_PLACEMENT_3D('',#24818,#20869,#20870);
#18382=AXIS2_PLACEMENT_3D('',#24820,#20872,#20873);
#18383=AXIS2_PLACEMENT_3D('',#24822,#20875,#20876);
#18384=AXIS2_PLACEMENT_3D('',#24823,#20877,#20878);
#18385=AXIS2_PLACEMENT_3D('',#24825,#20880,#20881);
#18386=AXIS2_PLACEMENT_3D('',#24827,#20883,#20884);
#18387=AXIS2_PLACEMENT_3D('',#24828,#20885,#20886);
#18388=AXIS2_PLACEMENT_3D('',#24830,#20888,#20889);
#18389=AXIS2_PLACEMENT_3D('',#24832,#20891,#20892);
#18390=AXIS2_PLACEMENT_3D('',#24833,#20893,#20894);
#18391=AXIS2_PLACEMENT_3D('',#24835,#20896,#20897);
#18392=AXIS2_PLACEMENT_3D('',#24837,#20899,#20900);
#18393=AXIS2_PLACEMENT_3D('',#24838,#20901,#20902);
#19603=DIRECTION('axis',(0.,0.,1.));
#19604=DIRECTION('refdir',(1.,0.,0.));
#19605=DIRECTION('center_axis',(-1.,0.,0.));
#19606=DIRECTION('ref_axis',(0.,0.,1.));
#19607=DIRECTION('center_axis',(-1.,0.,0.));
#19608=DIRECTION('ref_axis',(0.,0.997668769190539,0.0682424133646747));
#19609=DIRECTION('center_axis',(-1.,0.,0.));
#19610=DIRECTION('ref_axis',(0.,0.997668769190539,0.0682424133646747));
#19611=DIRECTION('center_axis',(-1.,0.,0.));
#19612=DIRECTION('ref_axis',(0.,0.997668769190539,0.0682424133646747));
#19613=DIRECTION('center_axis',(-1.,0.,0.));
#19614=DIRECTION('ref_axis',(0.,0.,1.));
#19615=DIRECTION('center_axis',(-1.,0.,0.));
#19616=DIRECTION('ref_axis',(0.,0.979084087682322,0.203456013052637));
#19617=DIRECTION('center_axis',(-1.,0.,0.));
#19618=DIRECTION('ref_axis',(0.,0.979084087682322,0.203456013052637));
#19619=DIRECTION('center_axis',(-1.,0.,0.));
#19620=DIRECTION('ref_axis',(0.,0.979084087682322,0.203456013052637));
#19621=DIRECTION('center_axis',(-1.,0.,0.));
#19622=DIRECTION('ref_axis',(0.,0.,1.));
#19623=DIRECTION('center_axis',(-1.,0.,0.));
#19624=DIRECTION('ref_axis',(0.,0.942260922118819,0.33487961217099));
#19625=DIRECTION('center_axis',(-1.,0.,0.));
#19626=DIRECTION('ref_axis',(0.,0.942260922118819,0.33487961217099));
#19627=DIRECTION('center_axis',(-1.,0.,0.));
#19628=DIRECTION('ref_axis',(0.,0.942260922118819,0.33487961217099));
#19629=DIRECTION('center_axis',(-1.,0.,0.));
#19630=DIRECTION('ref_axis',(0.,0.,1.));
#19631=DIRECTION('center_axis',(-1.,0.,0.));
#19632=DIRECTION('ref_axis',(0.,0.887885218402373,0.460065037731156));
#19633=DIRECTION('center_axis',(-1.,0.,0.));
#19634=DIRECTION('ref_axis',(0.,0.887885218402373,0.460065037731156));
#19635=DIRECTION('center_axis',(-1.,0.,0.));
#19636=DIRECTION('ref_axis',(0.,0.887885218402373,0.460065037731156));
#19637=DIRECTION('center_axis',(-1.,0.,0.));
#19638=DIRECTION('ref_axis',(0.,0.,1.));
#19639=DIRECTION('center_axis',(-1.,0.,0.));
#19640=DIRECTION('ref_axis',(0.,0.816969893010439,0.576680322114871));
#19641=DIRECTION('center_axis',(-1.,0.,0.));
#19642=DIRECTION('ref_axis',(0.,0.816969893010439,0.576680322114871));
#19643=DIRECTION('center_axis',(-1.,0.,0.));
#19644=DIRECTION('ref_axis',(0.,0.816969893010439,0.576680322114871));
#19645=DIRECTION('center_axis',(-1.,0.,0.));
#19646=DIRECTION('ref_axis',(0.,0.,1.));
#19647=DIRECTION('center_axis',(-1.,0.,0.));
#19648=DIRECTION('ref_axis',(0.,0.730835964278121,0.682553143218658));
#19649=DIRECTION('center_axis',(-1.,0.,0.));
#19650=DIRECTION('ref_axis',(0.,0.730835964278121,0.682553143218658));
#19651=DIRECTION('center_axis',(-1.,0.,0.));
#19652=DIRECTION('ref_axis',(0.,0.730835964278121,0.682553143218658));
#19653=DIRECTION('center_axis',(-1.,0.,0.));
#19654=DIRECTION('ref_axis',(0.,0.,1.));
#19655=DIRECTION('center_axis',(-1.,0.,0.));
#19656=DIRECTION('ref_axis',(0.,0.631087944326049,0.775711290704423));
#19657=DIRECTION('center_axis',(-1.,0.,0.));
#19658=DIRECTION('ref_axis',(0.,0.631087944326049,0.775711290704423));
#19659=DIRECTION('center_axis',(-1.,0.,0.));
#19660=DIRECTION('ref_axis',(0.,0.631087944326049,0.775711290704423));
#19661=DIRECTION('center_axis',(-1.,0.,0.));
#19662=DIRECTION('ref_axis',(0.,0.,1.));
#19663=DIRECTION('center_axis',(-1.,0.,0.));
#19664=DIRECTION('ref_axis',(0.,0.519583950035429,0.854419404546491));
#19665=DIRECTION('center_axis',(-1.,0.,0.));
#19666=DIRECTION('ref_axis',(0.,0.519583950035429,0.854419404546491));
#19667=DIRECTION('center_axis',(-1.,0.,0.));
#19668=DIRECTION('ref_axis',(0.,0.519583950035429,0.854419404546491));
#19669=DIRECTION('center_axis',(-1.,0.,0.));
#19670=DIRECTION('ref_axis',(0.,0.,1.));
#19671=DIRECTION('center_axis',(-1.,0.,0.));
#19672=DIRECTION('ref_axis',(0.,0.398401089846236,0.917211301505455));
#19673=DIRECTION('center_axis',(-1.,0.,0.));
#19674=DIRECTION('ref_axis',(0.,0.398401089846236,0.917211301505455));
#19675=DIRECTION('center_axis',(-1.,0.,0.));
#19676=DIRECTION('ref_axis',(0.,0.398401089846236,0.917211301505455));
#19677=DIRECTION('center_axis',(-1.,0.,0.));
#19678=DIRECTION('ref_axis',(0.,0.,1.));
#19679=DIRECTION('center_axis',(-1.,0.,0.));
#19680=DIRECTION('ref_axis',(0.,0.269796771157019,0.962917287347801));
#19681=DIRECTION('center_axis',(-1.,0.,0.));
#19682=DIRECTION('ref_axis',(0.,0.269796771157019,0.962917287347801));
#19683=DIRECTION('center_axis',(-1.,0.,0.));
#19684=DIRECTION('ref_axis',(0.,0.269796771157019,0.962917287347801));
#19685=DIRECTION('center_axis',(-1.,0.,0.));
#19686=DIRECTION('ref_axis',(0.,0.,1.));
#19687=DIRECTION('center_axis',(-1.,0.,0.));
#19688=DIRECTION('ref_axis',(0.,0.13616664909624,0.990685946036332));
#19689=DIRECTION('center_axis',(-1.,0.,0.));
#19690=DIRECTION('ref_axis',(0.,0.13616664909624,0.990685946036332));
#19691=DIRECTION('center_axis',(-1.,0.,0.));
#19692=DIRECTION('ref_axis',(0.,0.13616664909624,0.990685946036332));
#19693=DIRECTION('center_axis',(-1.,0.,0.));
#19694=DIRECTION('ref_axis',(0.,0.,1.));
#19695=DIRECTION('center_axis',(-1.,0.,0.));
#19696=DIRECTION('ref_axis',(0.,-6.98296267768627E-15,1.));
#19697=DIRECTION('center_axis',(-1.,0.,0.));
#19698=DIRECTION('ref_axis',(0.,-6.98296267768627E-15,1.));
#19699=DIRECTION('center_axis',(-1.,0.,0.));
#19700=DIRECTION('ref_axis',(0.,-6.98296267768627E-15,1.));
#19701=DIRECTION('center_axis',(-1.,0.,0.));
#19702=DIRECTION('ref_axis',(0.,0.,1.));
#19703=DIRECTION('center_axis',(-1.,0.,0.));
#19704=DIRECTION('ref_axis',(0.,-0.136166649096254,0.99068594603633));
#19705=DIRECTION('center_axis',(-1.,0.,0.));
#19706=DIRECTION('ref_axis',(0.,-0.136166649096254,0.99068594603633));
#19707=DIRECTION('center_axis',(-1.,0.,0.));
#19708=DIRECTION('ref_axis',(0.,-0.136166649096254,0.99068594603633));
#19709=DIRECTION('center_axis',(-1.,0.,0.));
#19710=DIRECTION('ref_axis',(0.,0.,1.));
#19711=DIRECTION('center_axis',(-1.,0.,0.));
#19712=DIRECTION('ref_axis',(0.,-0.269796771157031,0.962917287347797));
#19713=DIRECTION('center_axis',(-1.,0.,0.));
#19714=DIRECTION('ref_axis',(0.,-0.269796771157031,0.962917287347797));
#19715=DIRECTION('center_axis',(-1.,0.,0.));
#19716=DIRECTION('ref_axis',(0.,-0.269796771157031,0.962917287347797));
#19717=DIRECTION('center_axis',(-1.,0.,0.));
#19718=DIRECTION('ref_axis',(0.,0.,1.));
#19719=DIRECTION('center_axis',(-1.,0.,0.));
#19720=DIRECTION('ref_axis',(0.,-0.398401089846249,0.91721130150545));
#19721=DIRECTION('center_axis',(-1.,0.,0.));
#19722=DIRECTION('ref_axis',(0.,-0.398401089846249,0.91721130150545));
#19723=DIRECTION('center_axis',(-1.,0.,0.));
#19724=DIRECTION('ref_axis',(0.,-0.398401089846249,0.91721130150545));
#19725=DIRECTION('center_axis',(-1.,0.,0.));
#19726=DIRECTION('ref_axis',(0.,0.,1.));
#19727=DIRECTION('center_axis',(-1.,0.,0.));
#19728=DIRECTION('ref_axis',(0.,-0.51958395003544,0.854419404546485));
#19729=DIRECTION('center_axis',(-1.,0.,0.));
#19730=DIRECTION('ref_axis',(0.,-0.51958395003544,0.854419404546485));
#19731=DIRECTION('center_axis',(-1.,0.,0.));
#19732=DIRECTION('ref_axis',(0.,-0.51958395003544,0.854419404546485));
#19733=DIRECTION('center_axis',(-1.,0.,0.));
#19734=DIRECTION('ref_axis',(0.,0.,1.));
#19735=DIRECTION('center_axis',(-1.,0.,0.));
#19736=DIRECTION('ref_axis',(0.,-0.631087944326059,0.775711290704415));
#19737=DIRECTION('center_axis',(-1.,0.,0.));
#19738=DIRECTION('ref_axis',(0.,-0.631087944326059,0.775711290704415));
#19739=DIRECTION('center_axis',(-1.,0.,0.));
#19740=DIRECTION('ref_axis',(0.,-0.631087944326059,0.775711290704415));
#19741=DIRECTION('center_axis',(-1.,0.,0.));
#19742=DIRECTION('ref_axis',(0.,0.,1.));
#19743=DIRECTION('center_axis',(-1.,0.,0.));
#19744=DIRECTION('ref_axis',(0.,-0.73083596427813,0.682553143218648));
#19745=DIRECTION('center_axis',(-1.,0.,0.));
#19746=DIRECTION('ref_axis',(0.,-0.73083596427813,0.682553143218648));
#19747=DIRECTION('center_axis',(-1.,0.,0.));
#19748=DIRECTION('ref_axis',(0.,-0.73083596427813,0.682553143218648));
#19749=DIRECTION('center_axis',(-1.,0.,0.));
#19750=DIRECTION('ref_axis',(0.,0.,1.));
#19751=DIRECTION('center_axis',(-1.,0.,0.));
#19752=DIRECTION('ref_axis',(0.,-0.816969893010447,0.57668032211486));
#19753=DIRECTION('center_axis',(-1.,0.,0.));
#19754=DIRECTION('ref_axis',(0.,-0.816969893010447,0.57668032211486));
#19755=DIRECTION('center_axis',(-1.,0.,0.));
#19756=DIRECTION('ref_axis',(0.,-0.816969893010447,0.57668032211486));
#19757=DIRECTION('center_axis',(-1.,0.,0.));
#19758=DIRECTION('ref_axis',(0.,0.,1.));
#19759=DIRECTION('center_axis',(-1.,0.,0.));
#19760=DIRECTION('ref_axis',(0.,-0.887885218402379,0.460065037731144));
#19761=DIRECTION('center_axis',(-1.,0.,0.));
#19762=DIRECTION('ref_axis',(0.,-0.887885218402379,0.460065037731144));
#19763=DIRECTION('center_axis',(-1.,0.,0.));
#19764=DIRECTION('ref_axis',(0.,-0.887885218402379,0.460065037731144));
#19765=DIRECTION('center_axis',(-1.,0.,0.));
#19766=DIRECTION('ref_axis',(0.,0.,1.));
#19767=DIRECTION('center_axis',(-1.,0.,0.));
#19768=DIRECTION('ref_axis',(0.,-0.942260922118824,0.334879612170977));
#19769=DIRECTION('center_axis',(-1.,0.,0.));
#19770=DIRECTION('ref_axis',(0.,-0.942260922118824,0.334879612170977));
#19771=DIRECTION('center_axis',(-1.,0.,0.));
#19772=DIRECTION('ref_axis',(0.,-0.942260922118824,0.334879612170977));
#19773=DIRECTION('center_axis',(-1.,0.,0.));
#19774=DIRECTION('ref_axis',(0.,0.,1.));
#19775=DIRECTION('center_axis',(-1.,0.,0.));
#19776=DIRECTION('ref_axis',(0.,-0.979084087682325,0.203456013052624));
#19777=DIRECTION('center_axis',(-1.,0.,0.));
#19778=DIRECTION('ref_axis',(0.,-0.979084087682325,0.203456013052624));
#19779=DIRECTION('center_axis',(-1.,0.,0.));
#19780=DIRECTION('ref_axis',(0.,-0.979084087682325,0.203456013052624));
#19781=DIRECTION('center_axis',(-1.,0.,0.));
#19782=DIRECTION('ref_axis',(0.,0.,1.));
#19783=DIRECTION('center_axis',(-1.,0.,0.));
#19784=DIRECTION('ref_axis',(0.,-0.99766876919054,0.0682424133646607));
#19785=DIRECTION('center_axis',(-1.,0.,0.));
#19786=DIRECTION('ref_axis',(0.,-0.99766876919054,0.0682424133646607));
#19787=DIRECTION('center_axis',(-1.,0.,0.));
#19788=DIRECTION('ref_axis',(0.,-0.99766876919054,0.0682424133646607));
#19789=DIRECTION('center_axis',(-1.,0.,0.));
#19790=DIRECTION('ref_axis',(0.,0.,1.));
#19791=DIRECTION('center_axis',(-1.,0.,0.));
#19792=DIRECTION('ref_axis',(0.,-0.997668769190538,-0.0682424133646816));
#19793=DIRECTION('center_axis',(-1.,0.,0.));
#19794=DIRECTION('ref_axis',(0.,-0.997668769190538,-0.0682424133646816));
#19795=DIRECTION('center_axis',(-1.,0.,0.));
#19796=DIRECTION('ref_axis',(0.,-0.997668769190538,-0.0682424133646816));
#19797=DIRECTION('center_axis',(-1.,0.,0.));
#19798=DIRECTION('ref_axis',(0.,0.,1.));
#19799=DIRECTION('center_axis',(-1.,0.,0.));
#19800=DIRECTION('ref_axis',(0.,-0.979084087682321,-0.203456013052644));
#19801=DIRECTION('center_axis',(-1.,0.,0.));
#19802=DIRECTION('ref_axis',(0.,-0.979084087682321,-0.203456013052644));
#19803=DIRECTION('center_axis',(-1.,0.,0.));
#19804=DIRECTION('ref_axis',(0.,-0.979084087682321,-0.203456013052644));
#19805=DIRECTION('center_axis',(-1.,0.,0.));
#19806=DIRECTION('ref_axis',(0.,0.,1.));
#19807=DIRECTION('center_axis',(-1.,0.,0.));
#19808=DIRECTION('ref_axis',(0.,-0.942260922118817,-0.334879612170997));
#19809=DIRECTION('center_axis',(-1.,0.,0.));
#19810=DIRECTION('ref_axis',(0.,-0.942260922118817,-0.334879612170997));
#19811=DIRECTION('center_axis',(-1.,0.,0.));
#19812=DIRECTION('ref_axis',(0.,-0.942260922118817,-0.334879612170997));
#19813=DIRECTION('center_axis',(-1.,0.,0.));
#19814=DIRECTION('ref_axis',(0.,0.,1.));
#19815=DIRECTION('center_axis',(-1.,0.,0.));
#19816=DIRECTION('ref_axis',(0.,-0.88788521840237,-0.460065037731162));
#19817=DIRECTION('center_axis',(-1.,0.,0.));
#19818=DIRECTION('ref_axis',(0.,-0.88788521840237,-0.460065037731162));
#19819=DIRECTION('center_axis',(-1.,0.,0.));
#19820=DIRECTION('ref_axis',(0.,-0.88788521840237,-0.460065037731162));
#19821=DIRECTION('center_axis',(-1.,0.,0.));
#19822=DIRECTION('ref_axis',(0.,0.,1.));
#19823=DIRECTION('center_axis',(-1.,0.,0.));
#19824=DIRECTION('ref_axis',(0.,-0.816969893010436,-0.576680322114876));
#19825=DIRECTION('center_axis',(-1.,0.,0.));
#19826=DIRECTION('ref_axis',(0.,-0.816969893010436,-0.576680322114876));
#19827=DIRECTION('center_axis',(-1.,0.,0.));
#19828=DIRECTION('ref_axis',(0.,-0.816969893010436,-0.576680322114876));
#19829=DIRECTION('center_axis',(-1.,0.,0.));
#19830=DIRECTION('ref_axis',(0.,0.,1.));
#19831=DIRECTION('center_axis',(-1.,0.,0.));
#19832=DIRECTION('ref_axis',(0.,-0.730835964278116,-0.682553143218663));
#19833=DIRECTION('center_axis',(-1.,0.,0.));
#19834=DIRECTION('ref_axis',(0.,-0.730835964278116,-0.682553143218663));
#19835=DIRECTION('center_axis',(-1.,0.,0.));
#19836=DIRECTION('ref_axis',(0.,-0.730835964278116,-0.682553143218663));
#19837=DIRECTION('center_axis',(-1.,0.,0.));
#19838=DIRECTION('ref_axis',(0.,0.,1.));
#19839=DIRECTION('center_axis',(-1.,0.,0.));
#19840=DIRECTION('ref_axis',(0.,-0.631087944326043,-0.775711290704428));
#19841=DIRECTION('center_axis',(-1.,0.,0.));
#19842=DIRECTION('ref_axis',(0.,-0.631087944326043,-0.775711290704428));
#19843=DIRECTION('center_axis',(-1.,0.,0.));
#19844=DIRECTION('ref_axis',(0.,-0.631087944326043,-0.775711290704428));
#19845=DIRECTION('center_axis',(-1.,0.,0.));
#19846=DIRECTION('ref_axis',(0.,0.,1.));
#19847=DIRECTION('center_axis',(-1.,0.,0.));
#19848=DIRECTION('ref_axis',(0.,-0.519583950035423,-0.854419404546495));
#19849=DIRECTION('center_axis',(-1.,0.,0.));
#19850=DIRECTION('ref_axis',(0.,-0.519583950035423,-0.854419404546495));
#19851=DIRECTION('center_axis',(-1.,0.,0.));
#19852=DIRECTION('ref_axis',(0.,-0.519583950035423,-0.854419404546495));
#19853=DIRECTION('center_axis',(-1.,0.,0.));
#19854=DIRECTION('ref_axis',(0.,0.,1.));
#19855=DIRECTION('center_axis',(-1.,0.,0.));
#19856=DIRECTION('ref_axis',(0.,-0.398401089846229,-0.917211301505458));
#19857=DIRECTION('center_axis',(-1.,0.,0.));
#19858=DIRECTION('ref_axis',(0.,-0.398401089846229,-0.917211301505458));
#19859=DIRECTION('center_axis',(-1.,0.,0.));
#19860=DIRECTION('ref_axis',(0.,-0.398401089846229,-0.917211301505458));
#19861=DIRECTION('center_axis',(-1.,0.,0.));
#19862=DIRECTION('ref_axis',(0.,0.,1.));
#19863=DIRECTION('center_axis',(-1.,0.,0.));
#19864=DIRECTION('ref_axis',(0.,-0.269796771157012,-0.962917287347803));
#19865=DIRECTION('center_axis',(-1.,0.,0.));
#19866=DIRECTION('ref_axis',(0.,-0.269796771157012,-0.962917287347803));
#19867=DIRECTION('center_axis',(-1.,0.,0.));
#19868=DIRECTION('ref_axis',(0.,-0.269796771157012,-0.962917287347803));
#19869=DIRECTION('center_axis',(-1.,0.,0.));
#19870=DIRECTION('ref_axis',(0.,0.,1.));
#19871=DIRECTION('center_axis',(-1.,0.,0.));
#19872=DIRECTION('ref_axis',(0.,-0.136166649096233,-0.990685946036333));
#19873=DIRECTION('center_axis',(-1.,0.,0.));
#19874=DIRECTION('ref_axis',(0.,-0.136166649096233,-0.990685946036333));
#19875=DIRECTION('center_axis',(-1.,0.,0.));
#19876=DIRECTION('ref_axis',(0.,-0.136166649096233,-0.990685946036333));
#19877=DIRECTION('center_axis',(-1.,0.,0.));
#19878=DIRECTION('ref_axis',(0.,0.,1.));
#19879=DIRECTION('center_axis',(-1.,0.,0.));
#19880=DIRECTION('ref_axis',(0.,0.,-1.));
#19881=DIRECTION('center_axis',(-1.,0.,0.));
#19882=DIRECTION('ref_axis',(0.,0.,-1.));
#19883=DIRECTION('center_axis',(-1.,0.,0.));
#19884=DIRECTION('ref_axis',(0.,0.,-1.));
#19885=DIRECTION('center_axis',(-1.,0.,0.));
#19886=DIRECTION('ref_axis',(0.,0.,1.));
#19887=DIRECTION('center_axis',(-1.,0.,0.));
#19888=DIRECTION('ref_axis',(0.,0.136166649096247,-0.990685946036331));
#19889=DIRECTION('center_axis',(-1.,0.,0.));
#19890=DIRECTION('ref_axis',(0.,0.136166649096247,-0.990685946036331));
#19891=DIRECTION('center_axis',(-1.,0.,0.));
#19892=DIRECTION('ref_axis',(0.,0.136166649096247,-0.990685946036331));
#19893=DIRECTION('center_axis',(-1.,0.,0.));
#19894=DIRECTION('ref_axis',(0.,0.,1.));
#19895=DIRECTION('center_axis',(-1.,0.,0.));
#19896=DIRECTION('ref_axis',(0.,0.269796771157025,-0.962917287347799));
#19897=DIRECTION('center_axis',(-1.,0.,0.));
#19898=DIRECTION('ref_axis',(0.,0.269796771157025,-0.962917287347799));
#19899=DIRECTION('center_axis',(-1.,0.,0.));
#19900=DIRECTION('ref_axis',(0.,0.269796771157025,-0.962917287347799));
#19901=DIRECTION('center_axis',(-1.,0.,0.));
#19902=DIRECTION('ref_axis',(0.,0.,1.));
#19903=DIRECTION('center_axis',(-1.,0.,0.));
#19904=DIRECTION('ref_axis',(0.,0.398401089846243,-0.917211301505452));
#19905=DIRECTION('center_axis',(-1.,0.,0.));
#19906=DIRECTION('ref_axis',(0.,0.398401089846243,-0.917211301505452));
#19907=DIRECTION('center_axis',(-1.,0.,0.));
#19908=DIRECTION('ref_axis',(0.,0.398401089846243,-0.917211301505452));
#19909=DIRECTION('center_axis',(-1.,0.,0.));
#19910=DIRECTION('ref_axis',(0.,0.,1.));
#19911=DIRECTION('center_axis',(-1.,0.,0.));
#19912=DIRECTION('ref_axis',(0.,0.519583950035435,-0.854419404546488));
#19913=DIRECTION('center_axis',(-1.,0.,0.));
#19914=DIRECTION('ref_axis',(0.,0.519583950035435,-0.854419404546488));
#19915=DIRECTION('center_axis',(-1.,0.,0.));
#19916=DIRECTION('ref_axis',(0.,0.519583950035435,-0.854419404546488));
#19917=DIRECTION('center_axis',(-1.,0.,0.));
#19918=DIRECTION('ref_axis',(0.,0.,1.));
#19919=DIRECTION('center_axis',(-1.,0.,0.));
#19920=DIRECTION('ref_axis',(0.,0.631087944326054,-0.775711290704419));
#19921=DIRECTION('center_axis',(-1.,0.,0.));
#19922=DIRECTION('ref_axis',(0.,0.631087944326054,-0.775711290704419));
#19923=DIRECTION('center_axis',(-1.,0.,0.));
#19924=DIRECTION('ref_axis',(0.,0.631087944326054,-0.775711290704419));
#19925=DIRECTION('center_axis',(-1.,0.,0.));
#19926=DIRECTION('ref_axis',(0.,0.,1.));
#19927=DIRECTION('center_axis',(-1.,0.,0.));
#19928=DIRECTION('ref_axis',(0.,0.730835964278126,-0.682553143218653));
#19929=DIRECTION('center_axis',(-1.,0.,0.));
#19930=DIRECTION('ref_axis',(0.,0.730835964278126,-0.682553143218653));
#19931=DIRECTION('center_axis',(-1.,0.,0.));
#19932=DIRECTION('ref_axis',(0.,0.730835964278126,-0.682553143218653));
#19933=DIRECTION('center_axis',(-1.,0.,0.));
#19934=DIRECTION('ref_axis',(0.,0.,1.));
#19935=DIRECTION('center_axis',(-1.,0.,0.));
#19936=DIRECTION('ref_axis',(0.,0.816969893010443,-0.576680322114865));
#19937=DIRECTION('center_axis',(-1.,0.,0.));
#19938=DIRECTION('ref_axis',(0.,0.816969893010443,-0.576680322114865));
#19939=DIRECTION('center_axis',(-1.,0.,0.));
#19940=DIRECTION('ref_axis',(0.,0.816969893010443,-0.576680322114865));
#19941=DIRECTION('center_axis',(-1.,0.,0.));
#19942=DIRECTION('ref_axis',(0.,0.,1.));
#19943=DIRECTION('center_axis',(-1.,0.,0.));
#19944=DIRECTION('ref_axis',(0.,0.887885218402376,-0.46006503773115));
#19945=DIRECTION('center_axis',(-1.,0.,0.));
#19946=DIRECTION('ref_axis',(0.,0.887885218402376,-0.46006503773115));
#19947=DIRECTION('center_axis',(-1.,0.,0.));
#19948=DIRECTION('ref_axis',(0.,0.887885218402376,-0.46006503773115));
#19949=DIRECTION('center_axis',(-1.,0.,0.));
#19950=DIRECTION('ref_axis',(0.,0.,1.));
#19951=DIRECTION('center_axis',(-1.,0.,0.));
#19952=DIRECTION('ref_axis',(0.,0.942260922118822,-0.334879612170983));
#19953=DIRECTION('center_axis',(-1.,0.,0.));
#19954=DIRECTION('ref_axis',(0.,0.942260922118822,-0.334879612170983));
#19955=DIRECTION('center_axis',(-1.,0.,0.));
#19956=DIRECTION('ref_axis',(0.,0.942260922118822,-0.334879612170983));
#19957=DIRECTION('center_axis',(-1.,0.,0.));
#19958=DIRECTION('ref_axis',(0.,0.,1.));
#19959=DIRECTION('center_axis',(-1.,0.,0.));
#19960=DIRECTION('ref_axis',(0.,0.979084087682324,-0.203456013052631));
#19961=DIRECTION('center_axis',(-1.,0.,0.));
#19962=DIRECTION('ref_axis',(0.,0.979084087682323,-0.203456013052631));
#19963=DIRECTION('center_axis',(-1.,0.,0.));
#19964=DIRECTION('ref_axis',(0.,0.979084087682324,-0.203456013052631));
#19965=DIRECTION('center_axis',(-1.,0.,0.));
#19966=DIRECTION('ref_axis',(0.,0.,1.));
#19967=DIRECTION('center_axis',(-1.,0.,0.));
#19968=DIRECTION('ref_axis',(0.,0.997668769190539,-0.0682424133646677));
#19969=DIRECTION('center_axis',(-1.,0.,0.));
#19970=DIRECTION('ref_axis',(0.,0.997668769190539,-0.0682424133646677));
#19971=DIRECTION('center_axis',(-1.,0.,0.));
#19972=DIRECTION('ref_axis',(0.,0.997668769190539,-0.0682424133646677));
#19973=DIRECTION('center_axis',(-1.,0.,0.));
#19974=DIRECTION('ref_axis',(0.,0.,1.));
#19975=DIRECTION('center_axis',(-1.,0.,0.));
#19976=DIRECTION('ref_axis',(0.,0.,1.));
#19977=DIRECTION('center_axis',(-1.,0.,0.));
#19978=DIRECTION('ref_axis',(0.,0.,1.));
#19979=DIRECTION('',(-1.,0.,0.));
#19980=DIRECTION('',(-1.,0.,0.));
#19981=DIRECTION('center_axis',(-1.,0.,0.));
#19982=DIRECTION('ref_axis',(0.,0.,1.));
#19983=DIRECTION('center_axis',(-1.,0.,0.));
#19984=DIRECTION('ref_axis',(0.,0.,1.));
#19985=DIRECTION('',(-1.,0.,0.));
#19986=DIRECTION('center_axis',(-1.,0.,0.));
#19987=DIRECTION('ref_axis',(0.,0.,1.));
#19988=DIRECTION('',(-1.,0.,0.));
#19989=DIRECTION('center_axis',(-1.,0.,0.));
#19990=DIRECTION('ref_axis',(0.,0.,1.));
#19991=DIRECTION('',(-1.,0.,0.));
#19992=DIRECTION('',(-1.,0.,0.));
#19993=DIRECTION('center_axis',(-1.,0.,0.));
#19994=DIRECTION('ref_axis',(0.,0.,1.));
#19995=DIRECTION('center_axis',(-1.,0.,0.));
#19996=DIRECTION('ref_axis',(0.,0.,1.));
#19997=DIRECTION('',(-1.,0.,0.));
#19998=DIRECTION('',(-1.,0.,0.));
#19999=DIRECTION('center_axis',(-1.,0.,0.));
#20000=DIRECTION('ref_axis',(0.,0.,1.));
#20001=DIRECTION('center_axis',(-1.,0.,0.));
#20002=DIRECTION('ref_axis',(0.,0.,1.));
#20003=DIRECTION('',(-1.,0.,0.));
#20004=DIRECTION('',(-1.,0.,0.));
#20005=DIRECTION('center_axis',(-1.,0.,0.));
#20006=DIRECTION('ref_axis',(0.,0.,1.));
#20007=DIRECTION('center_axis',(-1.,0.,0.));
#20008=DIRECTION('ref_axis',(0.,0.,1.));
#20009=DIRECTION('',(-1.,0.,0.));
#20010=DIRECTION('center_axis',(-1.,0.,0.));
#20011=DIRECTION('ref_axis',(0.,0.,1.));
#20012=DIRECTION('',(-1.,0.,0.));
#20013=DIRECTION('center_axis',(-1.,0.,0.));
#20014=DIRECTION('ref_axis',(0.,0.,1.));
#20015=DIRECTION('',(-1.,0.,0.));
#20016=DIRECTION('center_axis',(-1.,0.,0.));
#20017=DIRECTION('ref_axis',(0.,0.,1.));
#20018=DIRECTION('',(-1.,0.,0.));
#20019=DIRECTION('center_axis',(-1.,0.,0.));
#20020=DIRECTION('ref_axis',(0.,0.,1.));
#20021=DIRECTION('',(-1.,0.,0.));
#20022=DIRECTION('',(-1.,0.,0.));
#20023=DIRECTION('center_axis',(-1.,0.,0.));
#20024=DIRECTION('ref_axis',(0.,0.,1.));
#20025=DIRECTION('center_axis',(-1.,0.,0.));
#20026=DIRECTION('ref_axis',(0.,0.,1.));
#20027=DIRECTION('',(-1.,0.,0.));
#20028=DIRECTION('center_axis',(-1.,0.,0.));
#20029=DIRECTION('ref_axis',(0.,0.,1.));
#20030=DIRECTION('',(-1.,0.,0.));
#20031=DIRECTION('center_axis',(-1.,0.,0.));
#20032=DIRECTION('ref_axis',(0.,0.,1.));
#20033=DIRECTION('',(-1.,0.,0.));
#20034=DIRECTION('',(-1.,0.,0.));
#20035=DIRECTION('center_axis',(-1.,0.,0.));
#20036=DIRECTION('ref_axis',(0.,0.,1.));
#20037=DIRECTION('center_axis',(-1.,0.,0.));
#20038=DIRECTION('ref_axis',(0.,0.,1.));
#20039=DIRECTION('',(-1.,0.,0.));
#20040=DIRECTION('',(-1.,0.,0.));
#20041=DIRECTION('center_axis',(-1.,0.,0.));
#20042=DIRECTION('ref_axis',(0.,0.,1.));
#20043=DIRECTION('center_axis',(-1.,0.,0.));
#20044=DIRECTION('ref_axis',(0.,0.,1.));
#20045=DIRECTION('',(-1.,0.,0.));
#20046=DIRECTION('',(-1.,0.,0.));
#20047=DIRECTION('center_axis',(-1.,0.,0.));
#20048=DIRECTION('ref_axis',(0.,0.,1.));
#20049=DIRECTION('center_axis',(-1.,0.,0.));
#20050=DIRECTION('ref_axis',(0.,0.,1.));
#20051=DIRECTION('',(-1.,0.,0.));
#20052=DIRECTION('',(-1.,0.,0.));
#20053=DIRECTION('center_axis',(-1.,0.,0.));
#20054=DIRECTION('ref_axis',(0.,0.,1.));
#20055=DIRECTION('center_axis',(-1.,0.,0.));
#20056=DIRECTION('ref_axis',(0.,0.,1.));
#20057=DIRECTION('',(-1.,0.,0.));
#20058=DIRECTION('center_axis',(-1.,0.,0.));
#20059=DIRECTION('ref_axis',(0.,0.,1.));
#20060=DIRECTION('',(-1.,0.,0.));
#20061=DIRECTION('center_axis',(-1.,0.,0.));
#20062=DIRECTION('ref_axis',(0.,0.,1.));
#20063=DIRECTION('',(-1.,0.,0.));
#20064=DIRECTION('',(-1.,0.,0.));
#20065=DIRECTION('center_axis',(-1.,0.,0.));
#20066=DIRECTION('ref_axis',(0.,0.,1.));
#20067=DIRECTION('center_axis',(-1.,0.,0.));
#20068=DIRECTION('ref_axis',(0.,0.,1.));
#20069=DIRECTION('',(-1.,0.,0.));
#20070=DIRECTION('',(-1.,0.,0.));
#20071=DIRECTION('center_axis',(-1.,0.,0.));
#20072=DIRECTION('ref_axis',(0.,0.,1.));
#20073=DIRECTION('center_axis',(-1.,0.,0.));
#20074=DIRECTION('ref_axis',(0.,0.,1.));
#20075=DIRECTION('',(-1.,0.,0.));
#20076=DIRECTION('',(-1.,0.,0.));
#20077=DIRECTION('center_axis',(-1.,0.,0.));
#20078=DIRECTION('ref_axis',(0.,0.,1.));
#20079=DIRECTION('center_axis',(-1.,0.,0.));
#20080=DIRECTION('ref_axis',(0.,0.,1.));
#20081=DIRECTION('',(-1.,0.,0.));
#20082=DIRECTION('center_axis',(-1.,0.,0.));
#20083=DIRECTION('ref_axis',(0.,0.,1.));
#20084=DIRECTION('',(-1.,0.,0.));
#20085=DIRECTION('center_axis',(-1.,0.,0.));
#20086=DIRECTION('ref_axis',(0.,0.,1.));
#20087=DIRECTION('',(-1.,0.,0.));
#20088=DIRECTION('center_axis',(-1.,0.,0.));
#20089=DIRECTION('ref_axis',(0.,0.,1.));
#20090=DIRECTION('',(-1.,0.,0.));
#20091=DIRECTION('center_axis',(-1.,0.,0.));
#20092=DIRECTION('ref_axis',(0.,0.,1.));
#20093=DIRECTION('',(-1.,0.,0.));
#20094=DIRECTION('',(-1.,0.,0.));
#20095=DIRECTION('center_axis',(-1.,0.,0.));
#20096=DIRECTION('ref_axis',(0.,0.,1.));
#20097=DIRECTION('center_axis',(-1.,0.,0.));
#20098=DIRECTION('ref_axis',(0.,0.,1.));
#20099=DIRECTION('',(-1.,0.,0.));
#20100=DIRECTION('center_axis',(-1.,0.,0.));
#20101=DIRECTION('ref_axis',(0.,0.,1.));
#20102=DIRECTION('',(-1.,0.,0.));
#20103=DIRECTION('center_axis',(-1.,0.,0.));
#20104=DIRECTION('ref_axis',(0.,0.,1.));
#20105=DIRECTION('',(-1.,0.,0.));
#20106=DIRECTION('',(-1.,0.,0.));
#20107=DIRECTION('center_axis',(-1.,0.,0.));
#20108=DIRECTION('ref_axis',(0.,0.,1.));
#20109=DIRECTION('center_axis',(-1.,0.,0.));
#20110=DIRECTION('ref_axis',(0.,0.,1.));
#20111=DIRECTION('',(-1.,0.,0.));
#20112=DIRECTION('',(-1.,0.,0.));
#20113=DIRECTION('center_axis',(-1.,0.,0.));
#20114=DIRECTION('ref_axis',(0.,0.,1.));
#20115=DIRECTION('center_axis',(-1.,0.,0.));
#20116=DIRECTION('ref_axis',(0.,0.,1.));
#20117=DIRECTION('',(-1.,0.,0.));
#20118=DIRECTION('',(-1.,0.,0.));
#20119=DIRECTION('center_axis',(-1.,0.,0.));
#20120=DIRECTION('ref_axis',(0.,0.,1.));
#20121=DIRECTION('center_axis',(-1.,0.,0.));
#20122=DIRECTION('ref_axis',(0.,1.05356763564868E-14,-1.));
#20123=DIRECTION('',(-1.,0.,0.));
#20124=DIRECTION('center_axis',(-1.,0.,0.));
#20125=DIRECTION('ref_axis',(0.,0.,1.));
#20126=DIRECTION('',(-1.,0.,0.));
#20127=DIRECTION('center_axis',(-1.,0.,0.));
#20128=DIRECTION('ref_axis',(0.,0.,1.));
#20129=DIRECTION('',(-1.,0.,0.));
#20130=DIRECTION('',(-1.,0.,0.));
#20131=DIRECTION('center_axis',(-1.,0.,0.));
#20132=DIRECTION('ref_axis',(0.,0.,1.));
#20133=DIRECTION('center_axis',(-1.,0.,0.));
#20134=DIRECTION('ref_axis',(0.,0.,1.));
#20135=DIRECTION('',(-1.,0.,0.));
#20136=DIRECTION('',(-1.,0.,0.));
#20137=DIRECTION('center_axis',(-1.,0.,0.));
#20138=DIRECTION('ref_axis',(0.,0.,1.));
#20139=DIRECTION('center_axis',(-1.,0.,0.));
#20140=DIRECTION('ref_axis',(0.,0.,1.));
#20141=DIRECTION('',(-1.,0.,0.));
#20142=DIRECTION('',(-1.,0.,0.));
#20143=DIRECTION('center_axis',(-1.,0.,0.));
#20144=DIRECTION('ref_axis',(0.,0.,1.));
#20145=DIRECTION('center_axis',(-1.,0.,0.));
#20146=DIRECTION('ref_axis',(0.,0.,1.));
#20147=DIRECTION('',(-1.,0.,0.));
#20148=DIRECTION('center_axis',(-1.,0.,0.));
#20149=DIRECTION('ref_axis',(0.,0.,1.));
#20150=DIRECTION('',(-1.,0.,0.));
#20151=DIRECTION('center_axis',(-1.,0.,0.));
#20152=DIRECTION('ref_axis',(0.,0.,1.));
#20153=DIRECTION('',(-1.,0.,0.));
#20154=DIRECTION('',(-1.,0.,0.));
#20155=DIRECTION('center_axis',(-1.,0.,0.));
#20156=DIRECTION('ref_axis',(0.,0.,1.));
#20157=DIRECTION('center_axis',(-1.,0.,0.));
#20158=DIRECTION('ref_axis',(0.,0.,1.));
#20159=DIRECTION('',(-1.,0.,0.));
#20160=DIRECTION('',(-1.,0.,0.));
#20161=DIRECTION('center_axis',(-1.,0.,0.));
#20162=DIRECTION('ref_axis',(0.,0.,1.));
#20163=DIRECTION('center_axis',(-1.,0.,0.));
#20164=DIRECTION('ref_axis',(0.,0.,1.));
#20165=DIRECTION('',(-1.,0.,0.));
#20166=DIRECTION('center_axis',(-1.,0.,0.));
#20167=DIRECTION('ref_axis',(0.,0.,1.));
#20168=DIRECTION('',(-1.,0.,0.));
#20169=DIRECTION('center_axis',(-1.,0.,0.));
#20170=DIRECTION('ref_axis',(0.,0.,1.));
#20171=DIRECTION('',(-1.,0.,0.));
#20172=DIRECTION('',(-1.,0.,0.));
#20173=DIRECTION('center_axis',(-1.,0.,0.));
#20174=DIRECTION('ref_axis',(0.,0.,1.));
#20175=DIRECTION('center_axis',(-1.,0.,0.));
#20176=DIRECTION('ref_axis',(0.,0.,1.));
#20177=DIRECTION('',(-1.,0.,0.));
#20178=DIRECTION('',(-1.,0.,0.));
#20179=DIRECTION('center_axis',(-1.,0.,0.));
#20180=DIRECTION('ref_axis',(0.,0.,1.));
#20181=DIRECTION('center_axis',(-1.,0.,0.));
#20182=DIRECTION('ref_axis',(0.,0.,1.));
#20183=DIRECTION('',(-1.,0.,0.));
#20184=DIRECTION('',(-1.,0.,0.));
#20185=DIRECTION('center_axis',(-1.,0.,0.));
#20186=DIRECTION('ref_axis',(0.,0.,1.));
#20187=DIRECTION('center_axis',(-1.,0.,0.));
#20188=DIRECTION('ref_axis',(0.,0.,1.));
#20189=DIRECTION('',(-1.,0.,0.));
#20190=DIRECTION('center_axis',(-1.,0.,0.));
#20191=DIRECTION('ref_axis',(0.,0.,1.));
#20192=DIRECTION('',(-1.,0.,0.));
#20193=DIRECTION('center_axis',(-1.,0.,0.));
#20194=DIRECTION('ref_axis',(0.,0.,1.));
#20195=DIRECTION('',(-1.,0.,0.));
#20196=DIRECTION('',(-1.,0.,0.));
#20197=DIRECTION('center_axis',(-1.,0.,0.));
#20198=DIRECTION('ref_axis',(0.,0.,1.));
#20199=DIRECTION('center_axis',(-1.,0.,0.));
#20200=DIRECTION('ref_axis',(0.,0.,1.));
#20201=DIRECTION('',(-1.,0.,0.));
#20202=DIRECTION('',(-1.,0.,0.));
#20203=DIRECTION('center_axis',(-1.,0.,0.));
#20204=DIRECTION('ref_axis',(0.,0.,1.));
#20205=DIRECTION('center_axis',(-1.,0.,0.));
#20206=DIRECTION('ref_axis',(0.,0.,1.));
#20207=DIRECTION('',(-1.,0.,0.));
#20208=DIRECTION('',(-1.,0.,0.));
#20209=DIRECTION('center_axis',(-1.,0.,0.));
#20210=DIRECTION('ref_axis',(0.,0.,1.));
#20211=DIRECTION('center_axis',(-1.,0.,0.));
#20212=DIRECTION('ref_axis',(0.,0.,1.));
#20213=DIRECTION('',(-1.,0.,0.));
#20214=DIRECTION('center_axis',(-1.,0.,0.));
#20215=DIRECTION('ref_axis',(0.,0.,1.));
#20216=DIRECTION('',(-1.,0.,0.));
#20217=DIRECTION('center_axis',(-1.,0.,0.));
#20218=DIRECTION('ref_axis',(0.,0.,1.));
#20219=DIRECTION('',(-1.,0.,0.));
#20220=DIRECTION('',(-1.,0.,0.));
#20221=DIRECTION('center_axis',(-1.,0.,0.));
#20222=DIRECTION('ref_axis',(0.,0.,1.));
#20223=DIRECTION('center_axis',(-1.,0.,0.));
#20224=DIRECTION('ref_axis',(0.,0.,1.));
#20225=DIRECTION('',(-1.,0.,0.));
#20226=DIRECTION('',(-1.,0.,0.));
#20227=DIRECTION('center_axis',(-1.,0.,0.));
#20228=DIRECTION('ref_axis',(0.,0.,1.));
#20229=DIRECTION('center_axis',(-1.,0.,0.));
#20230=DIRECTION('ref_axis',(0.,0.,1.));
#20231=DIRECTION('',(-1.,0.,0.));
#20232=DIRECTION('center_axis',(-1.,0.,0.));
#20233=DIRECTION('ref_axis',(0.,0.,1.));
#20234=DIRECTION('',(-1.,0.,0.));
#20235=DIRECTION('center_axis',(-1.,0.,0.));
#20236=DIRECTION('ref_axis',(0.,0.,1.));
#20237=DIRECTION('',(-1.,0.,0.));
#20238=DIRECTION('',(-1.,0.,0.));
#20239=DIRECTION('center_axis',(-1.,0.,0.));
#20240=DIRECTION('ref_axis',(0.,0.,1.));
#20241=DIRECTION('center_axis',(-1.,0.,0.));
#20242=DIRECTION('ref_axis',(0.,0.,1.));
#20243=DIRECTION('',(-1.,0.,0.));
#20244=DIRECTION('',(-1.,0.,0.));
#20245=DIRECTION('center_axis',(-1.,0.,0.));
#20246=DIRECTION('ref_axis',(0.,0.,1.));
#20247=DIRECTION('center_axis',(1.,0.,0.));
#20248=DIRECTION('ref_axis',(0.,0.,-1.));
#20249=DIRECTION('center_axis',(-1.,0.,0.));
#20250=DIRECTION('ref_axis',(0.,0.997668769190539,0.0682424133646747));
#20251=DIRECTION('center_axis',(1.,0.,0.));
#20252=DIRECTION('ref_axis',(0.,0.,-1.));
#20253=DIRECTION('center_axis',(-1.,0.,0.));
#20254=DIRECTION('ref_axis',(0.,0.997668769190539,-0.0682424133646677));
#20255=DIRECTION('center_axis',(-1.,0.,0.));
#20256=DIRECTION('ref_axis',(0.,0.997668769190539,-0.0682424133646677));
#20257=DIRECTION('center_axis',(1.,0.,0.));
#20258=DIRECTION('ref_axis',(0.,0.,-1.));
#20259=DIRECTION('center_axis',(-1.,0.,0.));
#20260=DIRECTION('ref_axis',(0.,0.979084087682323,-0.203456013052631));
#20261=DIRECTION('center_axis',(-1.,0.,0.));
#20262=DIRECTION('ref_axis',(0.,0.979084087682324,-0.203456013052631));
#20263=DIRECTION('center_axis',(1.,0.,0.));
#20264=DIRECTION('ref_axis',(0.,0.,-1.));
#20265=DIRECTION('center_axis',(-1.,0.,0.));
#20266=DIRECTION('ref_axis',(0.,0.942260922118822,-0.334879612170983));
#20267=DIRECTION('center_axis',(-1.,0.,0.));
#20268=DIRECTION('ref_axis',(0.,0.942260922118822,-0.334879612170983));
#20269=DIRECTION('center_axis',(1.,0.,0.));
#20270=DIRECTION('ref_axis',(0.,0.,-1.));
#20271=DIRECTION('center_axis',(-1.,0.,0.));
#20272=DIRECTION('ref_axis',(0.,0.887885218402376,-0.46006503773115));
#20273=DIRECTION('center_axis',(-1.,0.,0.));
#20274=DIRECTION('ref_axis',(0.,0.887885218402376,-0.46006503773115));
#20275=DIRECTION('center_axis',(1.,0.,0.));
#20276=DIRECTION('ref_axis',(0.,0.,-1.));
#20277=DIRECTION('center_axis',(-1.,0.,0.));
#20278=DIRECTION('ref_axis',(0.,0.816969893010443,-0.576680322114865));
#20279=DIRECTION('center_axis',(-1.,0.,0.));
#20280=DIRECTION('ref_axis',(0.,0.816969893010443,-0.576680322114865));
#20281=DIRECTION('center_axis',(1.,0.,0.));
#20282=DIRECTION('ref_axis',(0.,0.,-1.));
#20283=DIRECTION('center_axis',(-1.,0.,0.));
#20284=DIRECTION('ref_axis',(0.,0.730835964278126,-0.682553143218653));
#20285=DIRECTION('center_axis',(-1.,0.,0.));
#20286=DIRECTION('ref_axis',(0.,0.730835964278126,-0.682553143218653));
#20287=DIRECTION('center_axis',(1.,0.,0.));
#20288=DIRECTION('ref_axis',(0.,0.,-1.));
#20289=DIRECTION('center_axis',(-1.,0.,0.));
#20290=DIRECTION('ref_axis',(0.,0.631087944326054,-0.775711290704419));
#20291=DIRECTION('center_axis',(-1.,0.,0.));
#20292=DIRECTION('ref_axis',(0.,0.631087944326054,-0.775711290704419));
#20293=DIRECTION('center_axis',(1.,0.,0.));
#20294=DIRECTION('ref_axis',(0.,0.,-1.));
#20295=DIRECTION('center_axis',(-1.,0.,0.));
#20296=DIRECTION('ref_axis',(0.,0.519583950035435,-0.854419404546488));
#20297=DIRECTION('center_axis',(-1.,0.,0.));
#20298=DIRECTION('ref_axis',(0.,0.519583950035435,-0.854419404546488));
#20299=DIRECTION('center_axis',(1.,0.,0.));
#20300=DIRECTION('ref_axis',(0.,0.,-1.));
#20301=DIRECTION('center_axis',(-1.,0.,0.));
#20302=DIRECTION('ref_axis',(0.,0.398401089846243,-0.917211301505452));
#20303=DIRECTION('center_axis',(-1.,0.,0.));
#20304=DIRECTION('ref_axis',(0.,0.398401089846243,-0.917211301505452));
#20305=DIRECTION('center_axis',(1.,0.,0.));
#20306=DIRECTION('ref_axis',(0.,0.,-1.));
#20307=DIRECTION('center_axis',(-1.,0.,0.));
#20308=DIRECTION('ref_axis',(0.,0.269796771157025,-0.962917287347799));
#20309=DIRECTION('center_axis',(-1.,0.,0.));
#20310=DIRECTION('ref_axis',(0.,0.269796771157025,-0.962917287347799));
#20311=DIRECTION('center_axis',(1.,0.,0.));
#20312=DIRECTION('ref_axis',(0.,0.,-1.));
#20313=DIRECTION('center_axis',(-1.,0.,0.));
#20314=DIRECTION('ref_axis',(0.,0.136166649096247,-0.990685946036331));
#20315=DIRECTION('center_axis',(-1.,0.,0.));
#20316=DIRECTION('ref_axis',(0.,0.136166649096247,-0.990685946036331));
#20317=DIRECTION('center_axis',(-1.,0.,0.));
#20318=DIRECTION('ref_axis',(0.,0.,1.));
#20319=DIRECTION('center_axis',(1.,0.,0.));
#20320=DIRECTION('ref_axis',(0.,0.,-1.));
#20321=DIRECTION('center_axis',(-1.,0.,0.));
#20322=DIRECTION('ref_axis',(0.,0.,-1.));
#20323=DIRECTION('center_axis',(-1.,0.,0.));
#20324=DIRECTION('ref_axis',(0.,0.,-1.));
#20325=DIRECTION('center_axis',(1.,0.,0.));
#20326=DIRECTION('ref_axis',(0.,0.,-1.));
#20327=DIRECTION('center_axis',(-1.,0.,0.));
#20328=DIRECTION('ref_axis',(0.,-0.136166649096233,-0.990685946036333));
#20329=DIRECTION('center_axis',(-1.,0.,0.));
#20330=DIRECTION('ref_axis',(0.,-0.136166649096233,-0.990685946036333));
#20331=DIRECTION('center_axis',(1.,0.,0.));
#20332=DIRECTION('ref_axis',(0.,0.,-1.));
#20333=DIRECTION('center_axis',(-1.,0.,0.));
#20334=DIRECTION('ref_axis',(0.,-0.269796771157012,-0.962917287347803));
#20335=DIRECTION('center_axis',(-1.,0.,0.));
#20336=DIRECTION('ref_axis',(0.,-0.269796771157012,-0.962917287347803));
#20337=DIRECTION('center_axis',(1.,0.,0.));
#20338=DIRECTION('ref_axis',(0.,0.,-1.));
#20339=DIRECTION('center_axis',(-1.,0.,0.));
#20340=DIRECTION('ref_axis',(0.,-0.398401089846229,-0.917211301505458));
#20341=DIRECTION('center_axis',(-1.,0.,0.));
#20342=DIRECTION('ref_axis',(0.,-0.398401089846229,-0.917211301505458));
#20343=DIRECTION('center_axis',(1.,0.,0.));
#20344=DIRECTION('ref_axis',(0.,0.,-1.));
#20345=DIRECTION('center_axis',(-1.,0.,0.));
#20346=DIRECTION('ref_axis',(0.,-0.519583950035423,-0.854419404546495));
#20347=DIRECTION('center_axis',(-1.,0.,0.));
#20348=DIRECTION('ref_axis',(0.,-0.519583950035423,-0.854419404546495));
#20349=DIRECTION('center_axis',(1.,0.,0.));
#20350=DIRECTION('ref_axis',(0.,0.,-1.));
#20351=DIRECTION('center_axis',(-1.,0.,0.));
#20352=DIRECTION('ref_axis',(0.,-0.631087944326043,-0.775711290704428));
#20353=DIRECTION('center_axis',(-1.,0.,0.));
#20354=DIRECTION('ref_axis',(0.,-0.631087944326043,-0.775711290704428));
#20355=DIRECTION('center_axis',(1.,0.,0.));
#20356=DIRECTION('ref_axis',(0.,0.,-1.));
#20357=DIRECTION('center_axis',(-1.,0.,0.));
#20358=DIRECTION('ref_axis',(0.,-0.730835964278116,-0.682553143218663));
#20359=DIRECTION('center_axis',(-1.,0.,0.));
#20360=DIRECTION('ref_axis',(0.,-0.730835964278116,-0.682553143218663));
#20361=DIRECTION('center_axis',(1.,0.,0.));
#20362=DIRECTION('ref_axis',(0.,0.,-1.));
#20363=DIRECTION('center_axis',(-1.,0.,0.));
#20364=DIRECTION('ref_axis',(0.,-0.816969893010436,-0.576680322114876));
#20365=DIRECTION('center_axis',(-1.,0.,0.));
#20366=DIRECTION('ref_axis',(0.,-0.816969893010436,-0.576680322114876));
#20367=DIRECTION('center_axis',(1.,0.,0.));
#20368=DIRECTION('ref_axis',(0.,0.,-1.));
#20369=DIRECTION('center_axis',(-1.,0.,0.));
#20370=DIRECTION('ref_axis',(0.,-0.88788521840237,-0.460065037731162));
#20371=DIRECTION('center_axis',(-1.,0.,0.));
#20372=DIRECTION('ref_axis',(0.,-0.88788521840237,-0.460065037731162));
#20373=DIRECTION('center_axis',(1.,0.,0.));
#20374=DIRECTION('ref_axis',(0.,0.,-1.));
#20375=DIRECTION('center_axis',(-1.,0.,0.));
#20376=DIRECTION('ref_axis',(0.,-0.942260922118817,-0.334879612170997));
#20377=DIRECTION('center_axis',(-1.,0.,0.));
#20378=DIRECTION('ref_axis',(0.,-0.942260922118817,-0.334879612170997));
#20379=DIRECTION('center_axis',(1.,0.,0.));
#20380=DIRECTION('ref_axis',(0.,0.,-1.));
#20381=DIRECTION('center_axis',(-1.,0.,0.));
#20382=DIRECTION('ref_axis',(0.,-0.979084087682321,-0.203456013052644));
#20383=DIRECTION('center_axis',(-1.,0.,0.));
#20384=DIRECTION('ref_axis',(0.,-0.979084087682321,-0.203456013052644));
#20385=DIRECTION('center_axis',(1.,0.,0.));
#20386=DIRECTION('ref_axis',(0.,0.,-1.));
#20387=DIRECTION('center_axis',(-1.,0.,0.));
#20388=DIRECTION('ref_axis',(0.,-0.997668769190538,-0.0682424133646816));
#20389=DIRECTION('center_axis',(-1.,0.,0.));
#20390=DIRECTION('ref_axis',(0.,-0.997668769190538,-0.0682424133646816));
#20391=DIRECTION('center_axis',(1.,0.,0.));
#20392=DIRECTION('ref_axis',(0.,0.,-1.));
#20393=DIRECTION('center_axis',(-1.,0.,0.));
#20394=DIRECTION('ref_axis',(0.,-0.99766876919054,0.0682424133646607));
#20395=DIRECTION('center_axis',(-1.,0.,0.));
#20396=DIRECTION('ref_axis',(0.,-0.99766876919054,0.0682424133646607));
#20397=DIRECTION('center_axis',(1.,0.,0.));
#20398=DIRECTION('ref_axis',(0.,0.,-1.));
#20399=DIRECTION('center_axis',(-1.,0.,0.));
#20400=DIRECTION('ref_axis',(0.,-0.979084087682325,0.203456013052624));
#20401=DIRECTION('center_axis',(-1.,0.,0.));
#20402=DIRECTION('ref_axis',(0.,-0.979084087682325,0.203456013052624));
#20403=DIRECTION('center_axis',(1.,0.,0.));
#20404=DIRECTION('ref_axis',(0.,0.,-1.));
#20405=DIRECTION('center_axis',(-1.,0.,0.));
#20406=DIRECTION('ref_axis',(0.,-0.942260922118824,0.334879612170977));
#20407=DIRECTION('center_axis',(-1.,0.,0.));
#20408=DIRECTION('ref_axis',(0.,-0.942260922118824,0.334879612170977));
#20409=DIRECTION('center_axis',(1.,0.,0.));
#20410=DIRECTION('ref_axis',(0.,0.,-1.));
#20411=DIRECTION('center_axis',(-1.,0.,0.));
#20412=DIRECTION('ref_axis',(0.,-0.887885218402379,0.460065037731144));
#20413=DIRECTION('center_axis',(-1.,0.,0.));
#20414=DIRECTION('ref_axis',(0.,-0.887885218402379,0.460065037731144));
#20415=DIRECTION('center_axis',(1.,0.,0.));
#20416=DIRECTION('ref_axis',(0.,0.,-1.));
#20417=DIRECTION('center_axis',(-1.,0.,0.));
#20418=DIRECTION('ref_axis',(0.,-0.816969893010447,0.57668032211486));
#20419=DIRECTION('center_axis',(-1.,0.,0.));
#20420=DIRECTION('ref_axis',(0.,-0.816969893010447,0.57668032211486));
#20421=DIRECTION('center_axis',(1.,0.,0.));
#20422=DIRECTION('ref_axis',(0.,0.,-1.));
#20423=DIRECTION('center_axis',(-1.,0.,0.));
#20424=DIRECTION('ref_axis',(0.,-0.73083596427813,0.682553143218648));
#20425=DIRECTION('center_axis',(-1.,0.,0.));
#20426=DIRECTION('ref_axis',(0.,-0.73083596427813,0.682553143218648));
#20427=DIRECTION('center_axis',(1.,0.,0.));
#20428=DIRECTION('ref_axis',(0.,0.,-1.));
#20429=DIRECTION('center_axis',(-1.,0.,0.));
#20430=DIRECTION('ref_axis',(0.,-0.631087944326059,0.775711290704415));
#20431=DIRECTION('center_axis',(-1.,0.,0.));
#20432=DIRECTION('ref_axis',(0.,-0.631087944326059,0.775711290704415));
#20433=DIRECTION('center_axis',(1.,0.,0.));
#20434=DIRECTION('ref_axis',(0.,0.,-1.));
#20435=DIRECTION('center_axis',(-1.,0.,0.));
#20436=DIRECTION('ref_axis',(0.,-0.51958395003544,0.854419404546485));
#20437=DIRECTION('center_axis',(-1.,0.,0.));
#20438=DIRECTION('ref_axis',(0.,-0.51958395003544,0.854419404546485));
#20439=DIRECTION('center_axis',(1.,0.,0.));
#20440=DIRECTION('ref_axis',(0.,0.,-1.));
#20441=DIRECTION('center_axis',(-1.,0.,0.));
#20442=DIRECTION('ref_axis',(0.,-0.398401089846249,0.91721130150545));
#20443=DIRECTION('center_axis',(-1.,0.,0.));
#20444=DIRECTION('ref_axis',(0.,-0.398401089846249,0.91721130150545));
#20445=DIRECTION('center_axis',(1.,0.,0.));
#20446=DIRECTION('ref_axis',(0.,0.,-1.));
#20447=DIRECTION('center_axis',(-1.,0.,0.));
#20448=DIRECTION('ref_axis',(0.,-0.269796771157031,0.962917287347797));
#20449=DIRECTION('center_axis',(-1.,0.,0.));
#20450=DIRECTION('ref_axis',(0.,-0.269796771157031,0.962917287347797));
#20451=DIRECTION('center_axis',(1.,0.,0.));
#20452=DIRECTION('ref_axis',(0.,0.,-1.));
#20453=DIRECTION('center_axis',(-1.,0.,0.));
#20454=DIRECTION('ref_axis',(0.,-0.136166649096254,0.99068594603633));
#20455=DIRECTION('center_axis',(-1.,0.,0.));
#20456=DIRECTION('ref_axis',(0.,-0.136166649096254,0.99068594603633));
#20457=DIRECTION('center_axis',(1.,0.,0.));
#20458=DIRECTION('ref_axis',(0.,0.,-1.));
#20459=DIRECTION('center_axis',(-1.,0.,0.));
#20460=DIRECTION('ref_axis',(0.,-6.98296267768627E-15,1.));
#20461=DIRECTION('center_axis',(-1.,0.,0.));
#20462=DIRECTION('ref_axis',(0.,-6.98296267768627E-15,1.));
#20463=DIRECTION('center_axis',(1.,0.,0.));
#20464=DIRECTION('ref_axis',(0.,0.,-1.));
#20465=DIRECTION('center_axis',(-1.,0.,0.));
#20466=DIRECTION('ref_axis',(0.,0.13616664909624,0.990685946036332));
#20467=DIRECTION('center_axis',(-1.,0.,0.));
#20468=DIRECTION('ref_axis',(0.,0.13616664909624,0.990685946036332));
#20469=DIRECTION('center_axis',(1.,0.,0.));
#20470=DIRECTION('ref_axis',(0.,0.,-1.));
#20471=DIRECTION('center_axis',(-1.,0.,0.));
#20472=DIRECTION('ref_axis',(0.,0.269796771157019,0.962917287347801));
#20473=DIRECTION('center_axis',(-1.,0.,0.));
#20474=DIRECTION('ref_axis',(0.,0.269796771157019,0.962917287347801));
#20475=DIRECTION('center_axis',(1.,0.,0.));
#20476=DIRECTION('ref_axis',(0.,0.,-1.));
#20477=DIRECTION('center_axis',(-1.,0.,0.));
#20478=DIRECTION('ref_axis',(0.,0.398401089846236,0.917211301505455));
#20479=DIRECTION('center_axis',(-1.,0.,0.));
#20480=DIRECTION('ref_axis',(0.,0.398401089846236,0.917211301505455));
#20481=DIRECTION('center_axis',(1.,0.,0.));
#20482=DIRECTION('ref_axis',(0.,0.,-1.));
#20483=DIRECTION('center_axis',(-1.,0.,0.));
#20484=DIRECTION('ref_axis',(0.,0.519583950035429,0.854419404546491));
#20485=DIRECTION('center_axis',(-1.,0.,0.));
#20486=DIRECTION('ref_axis',(0.,0.519583950035429,0.854419404546491));
#20487=DIRECTION('center_axis',(1.,0.,0.));
#20488=DIRECTION('ref_axis',(0.,0.,-1.));
#20489=DIRECTION('center_axis',(-1.,0.,0.));
#20490=DIRECTION('ref_axis',(0.,0.631087944326049,0.775711290704423));
#20491=DIRECTION('center_axis',(-1.,0.,0.));
#20492=DIRECTION('ref_axis',(0.,0.631087944326049,0.775711290704423));
#20493=DIRECTION('center_axis',(1.,0.,0.));
#20494=DIRECTION('ref_axis',(0.,0.,-1.));
#20495=DIRECTION('center_axis',(-1.,0.,0.));
#20496=DIRECTION('ref_axis',(0.,0.730835964278121,0.682553143218658));
#20497=DIRECTION('center_axis',(-1.,0.,0.));
#20498=DIRECTION('ref_axis',(0.,0.730835964278121,0.682553143218658));
#20499=DIRECTION('center_axis',(1.,0.,0.));
#20500=DIRECTION('ref_axis',(0.,0.,-1.));
#20501=DIRECTION('center_axis',(-1.,0.,0.));
#20502=DIRECTION('ref_axis',(0.,0.816969893010439,0.576680322114871));
#20503=DIRECTION('center_axis',(-1.,0.,0.));
#20504=DIRECTION('ref_axis',(0.,0.816969893010439,0.576680322114871));
#20505=DIRECTION('center_axis',(1.,0.,0.));
#20506=DIRECTION('ref_axis',(0.,0.,-1.));
#20507=DIRECTION('center_axis',(-1.,0.,0.));
#20508=DIRECTION('ref_axis',(0.,0.887885218402373,0.460065037731156));
#20509=DIRECTION('center_axis',(-1.,0.,0.));
#20510=DIRECTION('ref_axis',(0.,0.887885218402373,0.460065037731156));
#20511=DIRECTION('center_axis',(1.,0.,0.));
#20512=DIRECTION('ref_axis',(0.,0.,-1.));
#20513=DIRECTION('center_axis',(-1.,0.,0.));
#20514=DIRECTION('ref_axis',(0.,0.942260922118819,0.33487961217099));
#20515=DIRECTION('center_axis',(-1.,0.,0.));
#20516=DIRECTION('ref_axis',(0.,0.942260922118819,0.33487961217099));
#20517=DIRECTION('center_axis',(1.,0.,0.));
#20518=DIRECTION('ref_axis',(0.,0.,-1.));
#20519=DIRECTION('center_axis',(-1.,0.,0.));
#20520=DIRECTION('ref_axis',(0.,0.979084087682322,0.203456013052637));
#20521=DIRECTION('center_axis',(-1.,0.,0.));
#20522=DIRECTION('ref_axis',(0.,0.979084087682322,0.203456013052637));
#20523=DIRECTION('center_axis',(1.,0.,0.));
#20524=DIRECTION('ref_axis',(0.,0.,-1.));
#20525=DIRECTION('center_axis',(-1.,0.,0.));
#20526=DIRECTION('ref_axis',(0.,0.997668769190539,0.0682424133646747));
#20527=DIRECTION('center_axis',(1.,0.,0.));
#20528=DIRECTION('ref_axis',(0.,0.,-1.));
#20529=DIRECTION('center_axis',(-1.,0.,0.));
#20530=DIRECTION('ref_axis',(0.,0.,1.));
#20531=DIRECTION('',(-1.,0.,0.));
#20532=DIRECTION('',(-1.,0.,0.));
#20533=DIRECTION('center_axis',(-1.,0.,0.));
#20534=DIRECTION('ref_axis',(0.,0.,1.));
#20535=DIRECTION('',(-1.,0.,0.));
#20536=DIRECTION('center_axis',(-1.,0.,0.));
#20537=DIRECTION('ref_axis',(0.,0.,1.));
#20538=DIRECTION('',(-1.,0.,0.));
#20539=DIRECTION('center_axis',(-1.,0.,0.));
#20540=DIRECTION('ref_axis',(0.,0.,1.));
#20541=DIRECTION('center_axis',(-1.,0.,0.));
#20542=DIRECTION('ref_axis',(0.,0.,1.));
#20543=DIRECTION('',(-1.,0.,0.));
#20544=DIRECTION('center_axis',(-1.,0.,0.));
#20545=DIRECTION('ref_axis',(0.,0.,1.));
#20546=DIRECTION('',(-1.,0.,0.));
#20547=DIRECTION('center_axis',(-1.,0.,0.));
#20548=DIRECTION('ref_axis',(0.,0.,1.));
#20549=DIRECTION('center_axis',(-1.,0.,0.));
#20550=DIRECTION('ref_axis',(0.,0.,1.));
#20551=DIRECTION('',(-1.,0.,0.));
#20552=DIRECTION('center_axis',(-1.,0.,0.));
#20553=DIRECTION('ref_axis',(0.,0.,1.));
#20554=DIRECTION('',(-1.,0.,0.));
#20555=DIRECTION('center_axis',(-1.,0.,0.));
#20556=DIRECTION('ref_axis',(0.,0.,1.));
#20557=DIRECTION('center_axis',(-1.,0.,0.));
#20558=DIRECTION('ref_axis',(0.,0.,1.));
#20559=DIRECTION('',(-1.,0.,0.));
#20560=DIRECTION('center_axis',(-1.,0.,0.));
#20561=DIRECTION('ref_axis',(0.,0.,1.));
#20562=DIRECTION('',(-1.,0.,0.));
#20563=DIRECTION('center_axis',(-1.,0.,0.));
#20564=DIRECTION('ref_axis',(0.,0.,1.));
#20565=DIRECTION('center_axis',(-1.,0.,0.));
#20566=DIRECTION('ref_axis',(0.,0.,1.));
#20567=DIRECTION('',(-1.,0.,0.));
#20568=DIRECTION('center_axis',(-1.,0.,0.));
#20569=DIRECTION('ref_axis',(0.,0.,1.));
#20570=DIRECTION('',(-1.,0.,0.));
#20571=DIRECTION('center_axis',(-1.,0.,0.));
#20572=DIRECTION('ref_axis',(0.,0.,1.));
#20573=DIRECTION('center_axis',(-1.,0.,0.));
#20574=DIRECTION('ref_axis',(0.,0.,1.));
#20575=DIRECTION('',(-1.,0.,0.));
#20576=DIRECTION('center_axis',(-1.,0.,0.));
#20577=DIRECTION('ref_axis',(0.,0.,1.));
#20578=DIRECTION('',(-1.,0.,0.));
#20579=DIRECTION('center_axis',(-1.,0.,0.));
#20580=DIRECTION('ref_axis',(0.,0.,1.));
#20581=DIRECTION('center_axis',(-1.,0.,0.));
#20582=DIRECTION('ref_axis',(0.,0.,1.));
#20583=DIRECTION('',(-1.,0.,0.));
#20584=DIRECTION('center_axis',(-1.,0.,0.));
#20585=DIRECTION('ref_axis',(0.,0.,1.));
#20586=DIRECTION('',(-1.,0.,0.));
#20587=DIRECTION('center_axis',(-1.,0.,0.));
#20588=DIRECTION('ref_axis',(0.,0.,1.));
#20589=DIRECTION('center_axis',(-1.,0.,0.));
#20590=DIRECTION('ref_axis',(0.,0.,1.));
#20591=DIRECTION('',(-1.,0.,0.));
#20592=DIRECTION('center_axis',(-1.,0.,0.));
#20593=DIRECTION('ref_axis',(0.,0.,1.));
#20594=DIRECTION('',(-1.,0.,0.));
#20595=DIRECTION('center_axis',(-1.,0.,0.));
#20596=DIRECTION('ref_axis',(0.,0.,1.));
#20597=DIRECTION('center_axis',(-1.,0.,0.));
#20598=DIRECTION('ref_axis',(0.,0.,1.));
#20599=DIRECTION('',(-1.,0.,0.));
#20600=DIRECTION('center_axis',(-1.,0.,0.));
#20601=DIRECTION('ref_axis',(0.,0.,1.));
#20602=DIRECTION('',(-1.,0.,0.));
#20603=DIRECTION('center_axis',(-1.,0.,0.));
#20604=DIRECTION('ref_axis',(0.,0.,1.));
#20605=DIRECTION('center_axis',(-1.,0.,0.));
#20606=DIRECTION('ref_axis',(0.,0.,1.));
#20607=DIRECTION('',(-1.,0.,0.));
#20608=DIRECTION('center_axis',(-1.,0.,0.));
#20609=DIRECTION('ref_axis',(0.,0.,1.));
#20610=DIRECTION('',(-1.,0.,0.));
#20611=DIRECTION('center_axis',(-1.,0.,0.));
#20612=DIRECTION('ref_axis',(0.,0.,1.));
#20613=DIRECTION('center_axis',(-1.,0.,0.));
#20614=DIRECTION('ref_axis',(0.,0.,1.));
#20615=DIRECTION('',(-1.,0.,0.));
#20616=DIRECTION('center_axis',(-1.,0.,0.));
#20617=DIRECTION('ref_axis',(0.,-0.0311419921241395,-0.99951497053648));
#20618=DIRECTION('',(-1.,0.,0.));
#20619=DIRECTION('center_axis',(-1.,0.,0.));
#20620=DIRECTION('ref_axis',(0.,0.,1.));
#20621=DIRECTION('center_axis',(-1.,0.,0.));
#20622=DIRECTION('ref_axis',(0.,0.,1.));
#20623=DIRECTION('',(-1.,0.,0.));
#20624=DIRECTION('center_axis',(-1.,0.,0.));
#20625=DIRECTION('ref_axis',(0.,0.105248670330541,-0.994445934877132));
#20626=DIRECTION('',(-1.,0.,0.));
#20627=DIRECTION('center_axis',(-1.,0.,0.));
#20628=DIRECTION('ref_axis',(0.,0.,1.));
#20629=DIRECTION('center_axis',(-1.,0.,0.));
#20630=DIRECTION('ref_axis',(0.,0.,1.));
#20631=DIRECTION('',(-1.,0.,0.));
#20632=DIRECTION('center_axis',(-1.,0.,0.));
#20633=DIRECTION('ref_axis',(0.,0.,1.));
#20634=DIRECTION('',(-1.,0.,0.));
#20635=DIRECTION('center_axis',(-1.,0.,0.));
#20636=DIRECTION('ref_axis',(0.,0.,1.));
#20637=DIRECTION('center_axis',(-1.,0.,0.));
#20638=DIRECTION('ref_axis',(0.,0.,1.));
#20639=DIRECTION('',(-1.,0.,0.));
#20640=DIRECTION('center_axis',(-1.,0.,0.));
#20641=DIRECTION('ref_axis',(0.,0.,1.));
#20642=DIRECTION('',(-1.,0.,0.));
#20643=DIRECTION('center_axis',(-1.,0.,0.));
#20644=DIRECTION('ref_axis',(0.,0.,1.));
#20645=DIRECTION('center_axis',(-1.,0.,0.));
#20646=DIRECTION('ref_axis',(0.,-0.105248670330508,-0.994445934877136));
#20647=DIRECTION('',(-1.,0.,0.));
#20648=DIRECTION('center_axis',(-1.,0.,0.));
#20649=DIRECTION('ref_axis',(0.,0.,1.));
#20650=DIRECTION('',(-1.,0.,0.));
#20651=DIRECTION('center_axis',(-1.,0.,0.));
#20652=DIRECTION('ref_axis',(0.,0.,1.));
#20653=DIRECTION('center_axis',(-1.,0.,0.));
#20654=DIRECTION('ref_axis',(0.,0.0311419921241608,-0.999514970536479));
#20655=DIRECTION('',(-1.,0.,0.));
#20656=DIRECTION('center_axis',(-1.,0.,0.));
#20657=DIRECTION('ref_axis',(0.,0.,1.));
#20658=DIRECTION('',(-1.,0.,0.));
#20659=DIRECTION('center_axis',(-1.,0.,0.));
#20660=DIRECTION('ref_axis',(0.,0.,1.));
#20661=DIRECTION('center_axis',(-1.,0.,0.));
#20662=DIRECTION('ref_axis',(0.,0.,1.));
#20663=DIRECTION('',(-1.,0.,0.));
#20664=DIRECTION('center_axis',(-1.,0.,0.));
#20665=DIRECTION('ref_axis',(0.,0.,1.));
#20666=DIRECTION('',(-1.,0.,0.));
#20667=DIRECTION('center_axis',(-1.,0.,0.));
#20668=DIRECTION('ref_axis',(0.,0.,1.));
#20669=DIRECTION('center_axis',(-1.,0.,0.));
#20670=DIRECTION('ref_axis',(0.,0.,1.));
#20671=DIRECTION('',(-1.,0.,0.));
#20672=DIRECTION('center_axis',(-1.,0.,0.));
#20673=DIRECTION('ref_axis',(0.,0.,1.));
#20674=DIRECTION('',(-1.,0.,0.));
#20675=DIRECTION('center_axis',(-1.,0.,0.));
#20676=DIRECTION('ref_axis',(0.,0.,1.));
#20677=DIRECTION('center_axis',(-1.,0.,0.));
#20678=DIRECTION('ref_axis',(0.,0.,1.));
#20679=DIRECTION('',(-1.,0.,0.));
#20680=DIRECTION('center_axis',(-1.,0.,0.));
#20681=DIRECTION('ref_axis',(0.,0.,1.));
#20682=DIRECTION('',(-1.,0.,0.));
#20683=DIRECTION('center_axis',(-1.,0.,0.));
#20684=DIRECTION('ref_axis',(0.,0.,1.));
#20685=DIRECTION('center_axis',(-1.,0.,0.));
#20686=DIRECTION('ref_axis',(0.,0.,1.));
#20687=DIRECTION('',(-1.,0.,0.));
#20688=DIRECTION('center_axis',(-1.,0.,0.));
#20689=DIRECTION('ref_axis',(0.,0.,1.));
#20690=DIRECTION('',(-1.,0.,0.));
#20691=DIRECTION('center_axis',(-1.,0.,0.));
#20692=DIRECTION('ref_axis',(0.,0.,1.));
#20693=DIRECTION('center_axis',(-1.,0.,0.));
#20694=DIRECTION('ref_axis',(0.,0.,1.));
#20695=DIRECTION('',(-1.,0.,0.));
#20696=DIRECTION('center_axis',(-1.,0.,0.));
#20697=DIRECTION('ref_axis',(0.,0.,1.));
#20698=DIRECTION('',(-1.,0.,0.));
#20699=DIRECTION('center_axis',(-1.,0.,0.));
#20700=DIRECTION('ref_axis',(0.,0.,1.));
#20701=DIRECTION('center_axis',(-1.,0.,0.));
#20702=DIRECTION('ref_axis',(0.,0.,1.));
#20703=DIRECTION('',(-1.,0.,0.));
#20704=DIRECTION('center_axis',(-1.,0.,0.));
#20705=DIRECTION('ref_axis',(0.,0.,1.));
#20706=DIRECTION('',(-1.,0.,0.));
#20707=DIRECTION('center_axis',(-1.,0.,0.));
#20708=DIRECTION('ref_axis',(0.,0.,1.));
#20709=DIRECTION('center_axis',(-1.,0.,0.));
#20710=DIRECTION('ref_axis',(0.,0.,1.));
#20711=DIRECTION('',(-1.,0.,0.));
#20712=DIRECTION('center_axis',(-1.,0.,0.));
#20713=DIRECTION('ref_axis',(0.,0.,1.));
#20714=DIRECTION('',(-1.,0.,0.));
#20715=DIRECTION('center_axis',(-1.,0.,0.));
#20716=DIRECTION('ref_axis',(0.,0.,1.));
#20717=DIRECTION('center_axis',(-1.,0.,0.));
#20718=DIRECTION('ref_axis',(0.,0.,1.));
#20719=DIRECTION('',(-1.,0.,0.));
#20720=DIRECTION('center_axis',(-1.,0.,0.));
#20721=DIRECTION('ref_axis',(0.,0.,1.));
#20722=DIRECTION('',(-1.,0.,0.));
#20723=DIRECTION('center_axis',(-1.,0.,0.));
#20724=DIRECTION('ref_axis',(0.,0.,1.));
#20725=DIRECTION('center_axis',(-1.,0.,0.));
#20726=DIRECTION('ref_axis',(0.,0.,1.));
#20727=DIRECTION('',(-1.,0.,0.));
#20728=DIRECTION('center_axis',(-1.,0.,0.));
#20729=DIRECTION('ref_axis',(0.,0.,1.));
#20730=DIRECTION('',(-1.,0.,0.));
#20731=DIRECTION('center_axis',(-1.,0.,0.));
#20732=DIRECTION('ref_axis',(0.,0.,1.));
#20733=DIRECTION('center_axis',(-1.,0.,0.));
#20734=DIRECTION('ref_axis',(0.,0.,1.));
#20735=DIRECTION('',(-1.,0.,0.));
#20736=DIRECTION('center_axis',(-1.,0.,0.));
#20737=DIRECTION('ref_axis',(0.,0.,1.));
#20738=DIRECTION('',(-1.,0.,0.));
#20739=DIRECTION('center_axis',(-1.,0.,0.));
#20740=DIRECTION('ref_axis',(0.,0.,1.));
#20741=DIRECTION('center_axis',(-1.,0.,0.));
#20742=DIRECTION('ref_axis',(0.,0.,1.));
#20743=DIRECTION('',(-1.,0.,0.));
#20744=DIRECTION('center_axis',(-1.,0.,0.));
#20745=DIRECTION('ref_axis',(0.,0.,1.));
#20746=DIRECTION('',(-1.,0.,0.));
#20747=DIRECTION('center_axis',(-1.,0.,0.));
#20748=DIRECTION('ref_axis',(0.,0.,1.));
#20749=DIRECTION('center_axis',(-1.,0.,0.));
#20750=DIRECTION('ref_axis',(0.,0.,1.));
#20751=DIRECTION('',(-1.,0.,0.));
#20752=DIRECTION('center_axis',(-1.,0.,0.));
#20753=DIRECTION('ref_axis',(0.,0.,1.));
#20754=DIRECTION('',(-1.,0.,0.));
#20755=DIRECTION('center_axis',(-1.,0.,0.));
#20756=DIRECTION('ref_axis',(0.,0.,1.));
#20757=DIRECTION('center_axis',(-1.,0.,0.));
#20758=DIRECTION('ref_axis',(0.,0.,1.));
#20759=DIRECTION('',(-1.,0.,0.));
#20760=DIRECTION('center_axis',(-1.,0.,0.));
#20761=DIRECTION('ref_axis',(0.,0.,1.));
#20762=DIRECTION('',(-1.,0.,0.));
#20763=DIRECTION('center_axis',(-1.,0.,0.));
#20764=DIRECTION('ref_axis',(0.,0.,1.));
#20765=DIRECTION('center_axis',(-1.,0.,0.));
#20766=DIRECTION('ref_axis',(0.,0.,1.));
#20767=DIRECTION('',(-1.,0.,0.));
#20768=DIRECTION('center_axis',(-1.,0.,0.));
#20769=DIRECTION('ref_axis',(0.,0.,1.));
#20770=DIRECTION('',(-1.,0.,0.));
#20771=DIRECTION('center_axis',(-1.,0.,0.));
#20772=DIRECTION('ref_axis',(0.,0.,1.));
#20773=DIRECTION('center_axis',(-1.,0.,0.));
#20774=DIRECTION('ref_axis',(0.,0.,1.));
#20775=DIRECTION('',(-1.,0.,0.));
#20776=DIRECTION('center_axis',(-1.,0.,0.));
#20777=DIRECTION('ref_axis',(0.,0.,1.));
#20778=DIRECTION('',(-1.,0.,0.));
#20779=DIRECTION('center_axis',(-1.,0.,0.));
#20780=DIRECTION('ref_axis',(0.,0.,1.));
#20781=DIRECTION('center_axis',(-1.,0.,0.));
#20782=DIRECTION('ref_axis',(0.,0.,1.));
#20783=DIRECTION('',(-1.,0.,0.));
#20784=DIRECTION('center_axis',(-1.,0.,0.));
#20785=DIRECTION('ref_axis',(0.,0.,1.));
#20786=DIRECTION('',(-1.,0.,0.));
#20787=DIRECTION('center_axis',(-1.,0.,0.));
#20788=DIRECTION('ref_axis',(0.,0.,1.));
#20789=DIRECTION('center_axis',(-1.,0.,0.));
#20790=DIRECTION('ref_axis',(0.,0.,1.));
#20791=DIRECTION('',(-1.,0.,0.));
#20792=DIRECTION('center_axis',(-1.,0.,0.));
#20793=DIRECTION('ref_axis',(0.,0.,1.));
#20794=DIRECTION('',(-1.,0.,0.));
#20795=DIRECTION('center_axis',(-1.,0.,0.));
#20796=DIRECTION('ref_axis',(0.,0.,1.));
#20797=DIRECTION('center_axis',(-1.,0.,0.));
#20798=DIRECTION('ref_axis',(0.,0.,1.));
#20799=DIRECTION('',(-1.,0.,0.));
#20800=DIRECTION('center_axis',(-1.,0.,0.));
#20801=DIRECTION('ref_axis',(0.,0.,1.));
#20802=DIRECTION('',(-1.,0.,0.));
#20803=DIRECTION('center_axis',(-1.,0.,0.));
#20804=DIRECTION('ref_axis',(0.,0.,1.));
#20805=DIRECTION('center_axis',(-1.,0.,0.));
#20806=DIRECTION('ref_axis',(0.,0.,1.));
#20807=DIRECTION('',(-1.,0.,0.));
#20808=DIRECTION('center_axis',(-1.,0.,0.));
#20809=DIRECTION('ref_axis',(0.,0.,1.));
#20810=DIRECTION('',(-1.,0.,0.));
#20811=DIRECTION('center_axis',(-1.,0.,0.));
#20812=DIRECTION('ref_axis',(0.,0.,1.));
#20813=DIRECTION('center_axis',(-1.,0.,0.));
#20814=DIRECTION('ref_axis',(0.,0.,1.));
#20815=DIRECTION('',(-1.,0.,0.));
#20816=DIRECTION('center_axis',(-1.,0.,0.));
#20817=DIRECTION('ref_axis',(0.,0.,1.));
#20818=DIRECTION('',(-1.,0.,0.));
#20819=DIRECTION('center_axis',(-1.,0.,0.));
#20820=DIRECTION('ref_axis',(0.,0.,1.));
#20821=DIRECTION('center_axis',(-1.,0.,0.));
#20822=DIRECTION('ref_axis',(0.,0.,1.));
#20823=DIRECTION('',(-1.,0.,0.));
#20824=DIRECTION('center_axis',(-1.,0.,0.));
#20825=DIRECTION('ref_axis',(0.,0.,1.));
#20826=DIRECTION('',(-1.,0.,0.));
#20827=DIRECTION('center_axis',(-1.,0.,0.));
#20828=DIRECTION('ref_axis',(0.,0.,1.));
#20829=DIRECTION('center_axis',(-1.,0.,0.));
#20830=DIRECTION('ref_axis',(0.,0.,1.));
#20831=DIRECTION('',(-1.,0.,0.));
#20832=DIRECTION('center_axis',(-1.,0.,0.));
#20833=DIRECTION('ref_axis',(0.,0.,1.));
#20834=DIRECTION('',(-1.,0.,0.));
#20835=DIRECTION('center_axis',(-1.,0.,0.));
#20836=DIRECTION('ref_axis',(0.,0.,1.));
#20837=DIRECTION('center_axis',(-1.,0.,0.));
#20838=DIRECTION('ref_axis',(0.,0.,1.));
#20839=DIRECTION('',(-1.,0.,0.));
#20840=DIRECTION('center_axis',(-1.,0.,0.));
#20841=DIRECTION('ref_axis',(0.,0.,1.));
#20842=DIRECTION('',(-1.,0.,0.));
#20843=DIRECTION('center_axis',(-1.,0.,0.));
#20844=DIRECTION('ref_axis',(0.,0.,1.));
#20845=DIRECTION('center_axis',(-1.,0.,0.));
#20846=DIRECTION('ref_axis',(0.,0.,1.));
#20847=DIRECTION('',(-1.,0.,0.));
#20848=DIRECTION('center_axis',(-1.,0.,0.));
#20849=DIRECTION('ref_axis',(0.,0.,1.));
#20850=DIRECTION('',(-1.,0.,0.));
#20851=DIRECTION('center_axis',(-1.,0.,0.));
#20852=DIRECTION('ref_axis',(0.,0.,1.));
#20853=DIRECTION('center_axis',(-1.,0.,0.));
#20854=DIRECTION('ref_axis',(0.,0.,1.));
#20855=DIRECTION('',(-1.,0.,0.));
#20856=DIRECTION('center_axis',(-1.,0.,0.));
#20857=DIRECTION('ref_axis',(0.,0.,1.));
#20858=DIRECTION('',(-1.,0.,0.));
#20859=DIRECTION('center_axis',(-1.,0.,0.));
#20860=DIRECTION('ref_axis',(0.,0.,1.));
#20861=DIRECTION('center_axis',(-1.,0.,0.));
#20862=DIRECTION('ref_axis',(0.,0.,1.));
#20863=DIRECTION('',(-1.,0.,0.));
#20864=DIRECTION('center_axis',(-1.,0.,0.));
#20865=DIRECTION('ref_axis',(0.,0.,1.));
#20866=DIRECTION('',(-1.,0.,0.));
#20867=DIRECTION('center_axis',(-1.,0.,0.));
#20868=DIRECTION('ref_axis',(0.,0.,1.));
#20869=DIRECTION('center_axis',(-1.,0.,0.));
#20870=DIRECTION('ref_axis',(0.,0.,1.));
#20871=DIRECTION('',(-1.,0.,0.));
#20872=DIRECTION('center_axis',(-1.,0.,0.));
#20873=DIRECTION('ref_axis',(0.,0.,1.));
#20874=DIRECTION('',(-1.,0.,0.));
#20875=DIRECTION('center_axis',(-1.,0.,0.));
#20876=DIRECTION('ref_axis',(0.,0.,1.));
#20877=DIRECTION('center_axis',(-1.,0.,0.));
#20878=DIRECTION('ref_axis',(0.,0.,1.));
#20879=DIRECTION('',(-1.,0.,0.));
#20880=DIRECTION('center_axis',(-1.,0.,0.));
#20881=DIRECTION('ref_axis',(0.,0.,1.));
#20882=DIRECTION('',(-1.,0.,0.));
#20883=DIRECTION('center_axis',(-1.,0.,0.));
#20884=DIRECTION('ref_axis',(0.,0.,1.));
#20885=DIRECTION('center_axis',(-1.,0.,0.));
#20886=DIRECTION('ref_axis',(0.,0.,1.));
#20887=DIRECTION('',(-1.,0.,0.));
#20888=DIRECTION('center_axis',(-1.,0.,0.));
#20889=DIRECTION('ref_axis',(0.,0.,1.));
#20890=DIRECTION('',(-1.,0.,0.));
#20891=DIRECTION('center_axis',(-1.,0.,0.));
#20892=DIRECTION('ref_axis',(0.,0.,1.));
#20893=DIRECTION('center_axis',(-1.,0.,0.));
#20894=DIRECTION('ref_axis',(0.,0.,1.));
#20895=DIRECTION('',(-1.,0.,0.));
#20896=DIRECTION('center_axis',(-1.,0.,0.));
#20897=DIRECTION('ref_axis',(0.,0.,1.));
#20898=DIRECTION('',(-1.,0.,0.));
#20899=DIRECTION('center_axis',(-1.,0.,0.));
#20900=DIRECTION('ref_axis',(0.,0.,1.));
#20901=DIRECTION('center_axis',(-1.,0.,0.));
#20902=DIRECTION('ref_axis',(0.,0.,1.));
#20903=DIRECTION('',(-1.,0.,0.));
#23727=CARTESIAN_POINT('',(0.,0.,0.));
#23728=CARTESIAN_POINT('Origin',(0.012,0.,0.));
#23729=CARTESIAN_POINT('',(0.012,-0.000521792360520078,0.0108614735985732));
#23730=CARTESIAN_POINT('',(0.012,-0.000157005585611549,0.011998972841293));
#23731=CARTESIAN_POINT('Origin',(0.012,0.00400379034671789,0.010037397655502));
#23732=CARTESIAN_POINT('',(0.012,-0.000962038105848782,0.0108313599646072));
#23733=CARTESIAN_POINT('Origin',(0.012,0.,0.));
#23734=CARTESIAN_POINT('',(0.012,-0.00147831669728126,0.0119085926852227));
#23735=CARTESIAN_POINT('Origin',(0.012,-0.00533325763176565,0.00939872607688738));
#23736=CARTESIAN_POINT('',(0.012,-0.0017894031515103,0.0118658348362585));
#23737=CARTESIAN_POINT('Origin',(0.012,0.,0.));
#23738=CARTESIAN_POINT('',(0.012,-0.00199590282248143,0.0106892585300951));
#23739=CARTESIAN_POINT('Origin',(0.012,0.00259974002297311,0.0104890915072804));
#23740=CARTESIAN_POINT('',(0.012,-0.0024279476225516,0.0105994785882205));
#23741=CARTESIAN_POINT('Origin',(0.012,0.,0.));
#23742=CARTESIAN_POINT('',(0.012,-0.00308610073718624,0.0115963779793493));
#23743=CARTESIAN_POINT('Origin',(0.012,-0.00656337641804451,0.008584974014533));
#23744=CARTESIAN_POINT('',(0.012,-0.00338846752237721,0.0115116587792461));
#23745=CARTESIAN_POINT('Origin',(0.012,0.,0.));
#23746=CARTESIAN_POINT('',(0.012,-0.00343283339125312,0.0103179228000551));
#23747=CARTESIAN_POINT('Origin',(0.012,0.00114726146149736,0.0107453934304013));
#23748=CARTESIAN_POINT('',(0.012,-0.0038486290688996,0.0101701489807191));
#23749=CARTESIAN_POINT('Origin',(0.012,0.,0.));
#23750=CARTESIAN_POINT('',(0.012,-0.00463639655948427,0.0110681446929105));
#23751=CARTESIAN_POINT('Origin',(0.012,-0.00767123192004028,0.00761130012968249));
#23752=CARTESIAN_POINT('',(0.012,-0.00492441115452898,0.0109430423000713));
#23753=CARTESIAN_POINT('Origin',(0.012,0.,0.));
#23754=CARTESIAN_POINT('',(0.012,-0.00480581676911598,0.0097543836905098));
#23755=CARTESIAN_POINT('Origin',(0.012,-0.000326588410304044,0.0108015290049791));
#23756=CARTESIAN_POINT('',(0.012,-0.00519761783757985,0.00955136874036762));
#23757=CARTESIAN_POINT('Origin',(0.012,0.,0.));
#23758=CARTESIAN_POINT('',(0.012,-0.00610032508627829,0.0103337328125767));
#23759=CARTESIAN_POINT('Origin',(0.012,-0.0086361868858939,0.00649584212454889));
#23760=CARTESIAN_POINT('',(0.012,-0.0063686223242156,0.0101705776478774));
#23761=CARTESIAN_POINT('Origin',(0.012,0.,0.));
#23762=CARTESIAN_POINT('',(0.012,-0.00608927687352473,0.00900913886881298));
#23763=CARTESIAN_POINT('Origin',(0.012,-0.00179435455795048,0.0106564525314718));
#23764=CARTESIAN_POINT('',(0.012,-0.0064497848202166,0.0087546645722668));
#23765=CARTESIAN_POINT('Origin',(0.012,0.,0.));
#23766=CARTESIAN_POINT('',(0.012,-0.00745061609897327,0.0094068230421179));
#23767=CARTESIAN_POINT('Origin',(0.012,-0.00944026603035641,0.00525937887124024));
#23768=CARTESIAN_POINT('',(0.012,-0.00769419810989828,0.00920865437757535));
#23769=CARTESIAN_POINT('Origin',(0.012,0.,0.));
#23770=CARTESIAN_POINT('',(0.012,-0.00725930527113401,0.00809607083593554));
#23771=CARTESIAN_POINT('Origin',(0.012,-0.00322869527523151,0.0103128665100857));
#23772=CARTESIAN_POINT('',(0.012,-0.00758180451511425,0.00779487756764615));
#23773=CARTESIAN_POINT('Origin',(0.012,0.,0.));
#23774=CARTESIAN_POINT('',(0.012,-0.00866211623085141,0.00830468195677719));
#23775=CARTESIAN_POINT('Origin',(0.012,-0.0100684908803427,0.00392494334068737));
#23776=CARTESIAN_POINT('',(0.012,-0.00887644554277545,0.00807519129966231));
#23777=CARTESIAN_POINT('Origin',(0.012,0.,0.));
#23778=CARTESIAN_POINT('',(0.012,-0.00829410654667511,0.00703218832173891));
#23779=CARTESIAN_POINT('Origin',(0.012,-0.00460289150846104,0.00977717129830948));
#23780=CARTESIAN_POINT('',(0.012,-0.00857258953722036,0.006689886742415));
#23781=CARTESIAN_POINT('Origin',(0.012,0.,0.));
#23782=CARTESIAN_POINT('',(0.012,-0.0097122575267021,0.0070478403596434));
#23783=CARTESIAN_POINT('Origin',(0.012,-0.0105091587955445,0.00251739354197548));
#23784=CARTESIAN_POINT('',(0.012,-0.00989334159007065,0.00679130268668526));
#23785=CARTESIAN_POINT('Origin',(0.012,0.,0.));
#23786=CARTESIAN_POINT('',(0.012,-0.0091744043103039,0.00583730944451955));
#23787=CARTESIAN_POINT('Origin',(0.012,-0.00589134458189312,0.00905934588436428));
#23788=CARTESIAN_POINT('',(0.012,-0.00940368343621036,0.00546027598492447));
#23789=CARTESIAN_POINT('Origin',(0.012,0.,0.));
#23790=CARTESIAN_POINT('',(0.012,-0.0105814778411273,0.00565971083163554));
#23791=CARTESIAN_POINT('Origin',(0.012,-0.0107540609664773,0.00106294946466809));
#23792=CARTESIAN_POINT('',(0.012,-0.010725943402464,0.0053809049542934));
#23793=CARTESIAN_POINT('Origin',(0.012,0.,0.));
#23794=CARTESIAN_POINT('',(0.012,-0.00988380028027131,0.00453369253696241));
#23795=CARTESIAN_POINT('Origin',(0.012,-0.00707005305261656,0.00817276199753406));
#23796=CARTESIAN_POINT('',(0.012,-0.0100596045052361,0.00412895061707371));
#23797=CARTESIAN_POINT('Origin',(0.012,0.,0.));
#23798=CARTESIAN_POINT('',(0.012,-0.0112535852442972,0.00416615159941843));
#23799=CARTESIAN_POINT('Origin',(0.012,-0.0107986353290695,-0.000411295349988447));
#23800=CARTESIAN_POINT('',(0.012,-0.0113587411835337,0.00387027114366622));
#23801=CARTESIAN_POINT('Origin',(0.012,0.,0.));
#23802=CARTESIAN_POINT('',(0.012,-0.0104090797518856,0.00314562151551737));
#23803=CARTESIAN_POINT('Origin',(0.012,-0.00811705981202384,0.00713393501814931));
#23804=CARTESIAN_POINT('',(0.012,-0.010528134175832,0.00272071071150145));
#23805=CARTESIAN_POINT('Origin',(0.012,0.,0.));
#23806=CARTESIAN_POINT('',(0.012,-0.0117160596469668,0.0025949848455657));
#23807=CARTESIAN_POINT('Origin',(0.012,-0.0106420515472837,-0.00187787851047538));
#23808=CARTESIAN_POINT('',(0.012,-0.0117799471079178,0.00228754150446676));
#23809=CARTESIAN_POINT('Origin',(0.012,0.,0.));
#23810=CARTESIAN_POINT('',(0.012,-0.0107404577624574,0.00169895351698271));
#23811=CARTESIAN_POINT('Origin',(0.012,-0.00901286110520009,0.00596221632729986));
#23812=CARTESIAN_POINT('',(0.012,-0.0108005446267269,0.00126178911315627));
#23813=CARTESIAN_POINT('Origin',(0.012,0.,0.));
#23814=CARTESIAN_POINT('',(0.012,-0.0119602860260496,0.000975478433939967));
#23815=CARTESIAN_POINT('Origin',(0.012,-0.0102872264807069,-0.00330948034739476));
#23816=CARTESIAN_POINT('',(0.012,-0.0119817149061973,0.000662199295233823));
#23817=CARTESIAN_POINT('Origin',(0.012,0.,0.));
#23818=CARTESIAN_POINT('',(0.012,-0.0108717613666412,0.000220637228970165));
#23819=CARTESIAN_POINT('Origin',(0.012,-0.00974076984897455,0.00467943282721932));
#23820=CARTESIAN_POINT('',(0.012,-0.0108717613666412,-0.000220637228970318));
#23821=CARTESIAN_POINT('Origin',(0.012,0.,0.));
#23822=CARTESIAN_POINT('',(0.012,-0.0119817149061973,-0.000662199295233991));
#23823=CARTESIAN_POINT('Origin',(0.012,-0.00974076984897448,-0.00467943282721946));
#23824=CARTESIAN_POINT('',(0.012,-0.0119602860260496,-0.000975478433940136));
#23825=CARTESIAN_POINT('Origin',(0.012,0.,0.));
#23826=CARTESIAN_POINT('',(0.012,-0.0108005446267269,-0.00126178911315643));
#23827=CARTESIAN_POINT('Origin',(0.012,-0.0102872264807069,0.00330948034739461));
#23828=CARTESIAN_POINT('',(0.012,-0.0107404577624574,-0.00169895351698286));
#23829=CARTESIAN_POINT('Origin',(0.012,0.,0.));
#23830=CARTESIAN_POINT('',(0.012,-0.0117799471079178,-0.00228754150446692));
#23831=CARTESIAN_POINT('Origin',(0.012,-0.0090128611052,-0.00596221632729998));
#23832=CARTESIAN_POINT('',(0.012,-0.0117160596469668,-0.00259498484556586));
#23833=CARTESIAN_POINT('Origin',(0.012,0.,0.));
#23834=CARTESIAN_POINT('',(0.012,-0.0105281341758319,-0.00272071071150159));
#23835=CARTESIAN_POINT('Origin',(0.012,-0.0106420515472838,0.00187787851047525));
#23836=CARTESIAN_POINT('',(0.012,-0.0104090797518855,-0.00314562151551751));
#23837=CARTESIAN_POINT('Origin',(0.012,0.,0.));
#23838=CARTESIAN_POINT('',(0.012,-0.0113587411835336,-0.00387027114366637));
#23839=CARTESIAN_POINT('Origin',(0.012,-0.00811705981202375,-0.00713393501814942));
#23840=CARTESIAN_POINT('',(0.012,-0.0112535852442971,-0.00416615159941858));
#23841=CARTESIAN_POINT('Origin',(0.012,0.,0.));
#23842=CARTESIAN_POINT('',(0.012,-0.010059604505236,-0.00412895061707385));
#23843=CARTESIAN_POINT('Origin',(0.012,-0.0107986353290695,0.0004112953499883));
#23844=CARTESIAN_POINT('',(0.012,-0.00988380028027125,-0.00453369253696255));
#23845=CARTESIAN_POINT('Origin',(0.012,0.,0.));
#23846=CARTESIAN_POINT('',(0.012,-0.0107259434024639,-0.00538090495429355));
#23847=CARTESIAN_POINT('Origin',(0.012,-0.00707005305261645,-0.00817276199753415));
#23848=CARTESIAN_POINT('',(0.012,-0.0105814778411272,-0.00565971083163568));
#23849=CARTESIAN_POINT('Origin',(0.012,0.,0.));
#23850=CARTESIAN_POINT('',(0.012,-0.00940368343621029,-0.0054602759849246));
#23851=CARTESIAN_POINT('Origin',(0.012,-0.0107540609664773,-0.00106294946466824));
#23852=CARTESIAN_POINT('',(0.012,-0.00917440431030382,-0.00583730944451968));
#23853=CARTESIAN_POINT('Origin',(0.012,0.,0.));
#23854=CARTESIAN_POINT('',(0.012,-0.00989334159007055,-0.00679130268668539));
#23855=CARTESIAN_POINT('Origin',(0.012,-0.00589134458189299,-0.00905934588436437));
#23856=CARTESIAN_POINT('',(0.012,-0.009712257526702,-0.00704784035964354));
#23857=CARTESIAN_POINT('Origin',(0.012,0.,0.));
#23858=CARTESIAN_POINT('',(0.012,-0.00857258953722027,-0.00668988674241512));
#23859=CARTESIAN_POINT('Origin',(0.012,-0.0105091587955444,-0.00251739354197563));
#23860=CARTESIAN_POINT('',(0.012,-0.00829410654667501,-0.00703218832173902));
#23861=CARTESIAN_POINT('Origin',(0.012,0.,0.));
#23862=CARTESIAN_POINT('',(0.012,-0.00887644554277533,-0.00807519129966243));
#23863=CARTESIAN_POINT('Origin',(0.012,-0.0046028915084609,-0.00977717129830955));
#23864=CARTESIAN_POINT('',(0.012,-0.00866211623085129,-0.00830468195677731));
#23865=CARTESIAN_POINT('Origin',(0.012,0.,0.));
#23866=CARTESIAN_POINT('',(0.012,-0.00758180451511414,-0.00779487756764626));
#23867=CARTESIAN_POINT('Origin',(0.012,-0.0100684908803426,-0.00392494334068751));
#23868=CARTESIAN_POINT('',(0.012,-0.0072593052711339,-0.00809607083593564));
#23869=CARTESIAN_POINT('Origin',(0.012,0.,0.));
#23870=CARTESIAN_POINT('',(0.012,-0.00769419810989815,-0.00920865437757546));
#23871=CARTESIAN_POINT('Origin',(0.012,-0.00322869527523136,-0.0103128665100857));
#23872=CARTESIAN_POINT('',(0.012,-0.00745061609897314,-0.009406823042118));
#23873=CARTESIAN_POINT('Origin',(0.012,0.,0.));
#23874=CARTESIAN_POINT('',(0.012,-0.00644978482021648,-0.00875466457226689));
#23875=CARTESIAN_POINT('Origin',(0.012,-0.00944026603035634,-0.00525937887124037));
#23876=CARTESIAN_POINT('',(0.012,-0.0060892768735246,-0.00900913886881307));
#23877=CARTESIAN_POINT('Origin',(0.012,0.,0.));
#23878=CARTESIAN_POINT('',(0.012,-0.00636862232421547,-0.0101705776478774));
#23879=CARTESIAN_POINT('Origin',(0.012,-0.00179435455795034,-0.0106564525314718));
#23880=CARTESIAN_POINT('',(0.012,-0.00610032508627815,-0.0103337328125767));
#23881=CARTESIAN_POINT('Origin',(0.012,0.,0.));
#23882=CARTESIAN_POINT('',(0.012,-0.00519761783757972,-0.00955136874036769));
#23883=CARTESIAN_POINT('Origin',(0.012,-0.00863618688589381,-0.00649584212454901));
#23884=CARTESIAN_POINT('',(0.012,-0.00480581676911584,-0.00975438369050987));
#23885=CARTESIAN_POINT('Origin',(0.012,0.,0.));
#23886=CARTESIAN_POINT('',(0.012,-0.00492441115452883,-0.0109430423000714));
#23887=CARTESIAN_POINT('Origin',(0.012,-0.000326588410303897,-0.0108015290049791));
#23888=CARTESIAN_POINT('',(0.012,-0.00463639655948412,-0.0110681446929105));
#23889=CARTESIAN_POINT('Origin',(0.012,0.,0.));
#23890=CARTESIAN_POINT('',(0.012,-0.00384862906889946,-0.0101701489807191));
#23891=CARTESIAN_POINT('Origin',(0.012,-0.00767123192004017,-0.00761130012968259));
#23892=CARTESIAN_POINT('',(0.012,-0.00343283339125298,-0.0103179228000552));
#23893=CARTESIAN_POINT('Origin',(0.012,0.,0.));
#23894=CARTESIAN_POINT('',(0.012,-0.00338846752237705,-0.0115116587792462));
#23895=CARTESIAN_POINT('Origin',(0.012,0.0011472614614975,-0.0107453934304013));
#23896=CARTESIAN_POINT('',(0.012,-0.00308610073718608,-0.0115963779793494));
#23897=CARTESIAN_POINT('Origin',(0.012,0.,0.));
#23898=CARTESIAN_POINT('',(0.012,-0.00242794762255145,-0.0105994785882206));
#23899=CARTESIAN_POINT('Origin',(0.012,-0.00656337641804439,-0.00858497401453309));
#23900=CARTESIAN_POINT('',(0.012,-0.00199590282248128,-0.0106892585300951));
#23901=CARTESIAN_POINT('Origin',(0.012,0.,0.));
#23902=CARTESIAN_POINT('',(0.012,-0.00178940315151014,-0.0118658348362585));
#23903=CARTESIAN_POINT('Origin',(0.012,0.00259974002297325,-0.0104890915072803));
#23904=CARTESIAN_POINT('',(0.012,-0.00147831669728109,-0.0119085926852227));
#23905=CARTESIAN_POINT('Origin',(0.012,0.,0.));
#23906=CARTESIAN_POINT('',(0.012,-0.00096203810584863,-0.0108313599646072));
#23907=CARTESIAN_POINT('Origin',(0.012,-0.00533325763176552,-0.00939872607688746));
#23908=CARTESIAN_POINT('',(0.012,-0.000521792360519925,-0.0108614735985732));
#23909=CARTESIAN_POINT('Origin',(0.012,0.,0.));
#23910=CARTESIAN_POINT('',(0.012,-0.000157005585611382,-0.011998972841293));
#23911=CARTESIAN_POINT('Origin',(0.012,0.00400379034671803,-0.010037397655502));
#23912=CARTESIAN_POINT('',(0.012,0.000157005585611632,-0.011998972841293));
#23913=CARTESIAN_POINT('Origin',(0.012,0.,0.));
#23914=CARTESIAN_POINT('',(0.012,0.000521792360520154,-0.0108614735985732));
#23915=CARTESIAN_POINT('Origin',(0.012,-0.00400379034671782,-0.0100373976555021));
#23916=CARTESIAN_POINT('',(0.012,0.000962038105848858,-0.0108313599646072));
#23917=CARTESIAN_POINT('Origin',(0.012,0.,0.));
#23918=CARTESIAN_POINT('',(0.012,0.00147831669728134,-0.0119085926852227));
#23919=CARTESIAN_POINT('Origin',(0.012,0.00533325763176572,-0.00939872607688735));
#23920=CARTESIAN_POINT('',(0.012,0.00178940315151039,-0.0118658348362584));
#23921=CARTESIAN_POINT('Origin',(0.012,0.,0.));
#23922=CARTESIAN_POINT('',(0.012,0.00199590282248151,-0.0106892585300951));
#23923=CARTESIAN_POINT('Origin',(0.012,-0.00259974002297304,-0.0104890915072804));
#23924=CARTESIAN_POINT('',(0.012,0.00242794762255167,-0.0105994785882205));
#23925=CARTESIAN_POINT('Origin',(0.012,0.,0.));
#23926=CARTESIAN_POINT('',(0.012,0.00308610073718632,-0.0115963779793493));
#23927=CARTESIAN_POINT('Origin',(0.012,0.00656337641804457,-0.00858497401453295));
#23928=CARTESIAN_POINT('',(0.012,0.00338846752237729,-0.0115116587792461));
#23929=CARTESIAN_POINT('Origin',(0.012,0.,0.));
#23930=CARTESIAN_POINT('',(0.012,0.00343283339125319,-0.0103179228000551));
#23931=CARTESIAN_POINT('Origin',(0.012,-0.00114726146149728,-0.0107453934304014));
#23932=CARTESIAN_POINT('',(0.012,0.00384862906889967,-0.010170148980719));
#23933=CARTESIAN_POINT('Origin',(0.012,0.,0.));
#23934=CARTESIAN_POINT('',(0.012,0.00463639655948435,-0.0110681446929104));
#23935=CARTESIAN_POINT('Origin',(0.012,0.00767123192004033,-0.00761130012968243));
#23936=CARTESIAN_POINT('',(0.012,0.00492441115452905,-0.0109430423000713));
#23937=CARTESIAN_POINT('Origin',(0.012,0.,0.));
#23938=CARTESIAN_POINT('',(0.012,0.00480581676911604,-0.00975438369050977));
#23939=CARTESIAN_POINT('Origin',(0.012,0.000326588410304114,-0.0108015290049791));
#23940=CARTESIAN_POINT('',(0.012,0.00519761783757991,-0.00955136874036759));
#23941=CARTESIAN_POINT('Origin',(0.012,0.,0.));
#23942=CARTESIAN_POINT('',(0.012,0.00610032508627836,-0.0103337328125766));
#23943=CARTESIAN_POINT('Origin',(0.012,0.00863618688589394,-0.00649584212454884));
#23944=CARTESIAN_POINT('',(0.012,0.00636862232421567,-0.0101705776478773));
#23945=CARTESIAN_POINT('Origin',(0.012,0.,0.));
#23946=CARTESIAN_POINT('',(0.012,0.00608927687352478,-0.00900913886881295));
#23947=CARTESIAN_POINT('Origin',(0.012,0.00179435455795055,-0.0106564525314718));
#23948=CARTESIAN_POINT('',(0.012,0.00644978482021666,-0.00875466457226676));
#23949=CARTESIAN_POINT('Origin',(0.012,0.,0.));
#23950=CARTESIAN_POINT('',(0.012,0.00745061609897333,-0.00940682304211785));
#23951=CARTESIAN_POINT('Origin',(0.012,0.00944026603035645,-0.00525937887124018));
#23952=CARTESIAN_POINT('',(0.012,0.00769419810989834,-0.0092086543775753));
#23953=CARTESIAN_POINT('Origin',(0.012,0.,0.));
#23954=CARTESIAN_POINT('',(0.012,0.00725930527113406,-0.00809607083593549));
#23955=CARTESIAN_POINT('Origin',(0.012,0.00322869527523158,-0.0103128665100857));
#23956=CARTESIAN_POINT('',(0.012,0.0075818045151143,-0.0077948775676461));
#23957=CARTESIAN_POINT('Origin',(0.012,0.,0.));
#23958=CARTESIAN_POINT('',(0.012,0.00866211623085146,-0.00830468195677713));
#23959=CARTESIAN_POINT('Origin',(0.012,0.0100684908803427,-0.0039249433406873));
#23960=CARTESIAN_POINT('',(0.012,0.0088764455427755,-0.00807519129966225));
#23961=CARTESIAN_POINT('Origin',(0.012,0.,0.));
#23962=CARTESIAN_POINT('',(0.012,0.00829410654667516,-0.00703218832173885));
#23963=CARTESIAN_POINT('Origin',(0.012,0.0046028915084611,-0.00977717129830945));
#23964=CARTESIAN_POINT('',(0.012,0.00857258953722041,-0.00668988674241494));
#23965=CARTESIAN_POINT('Origin',(0.012,0.,0.));
#23966=CARTESIAN_POINT('',(0.012,0.00971225752670214,-0.00704784035964334));
#23967=CARTESIAN_POINT('Origin',(0.012,0.0105091587955445,-0.00251739354197541));
#23968=CARTESIAN_POINT('',(0.012,0.00989334159007069,-0.00679130268668519));
#23969=CARTESIAN_POINT('Origin',(0.012,0.,0.));
#23970=CARTESIAN_POINT('',(0.012,0.00917440431030394,-0.00583730944451949));
#23971=CARTESIAN_POINT('Origin',(0.012,0.00589134458189318,-0.00905934588436424));
#23972=CARTESIAN_POINT('',(0.012,0.0094036834362104,-0.0054602759849244));
#23973=CARTESIAN_POINT('Origin',(0.012,0.,0.));
#23974=CARTESIAN_POINT('',(0.012,0.0105814778411273,-0.00565971083163546));
#23975=CARTESIAN_POINT('Origin',(0.012,0.0107540609664773,-0.00106294946466802));
#23976=CARTESIAN_POINT('',(0.012,0.010725943402464,-0.00538090495429333));
#23977=CARTESIAN_POINT('Origin',(0.012,0.,0.));
#23978=CARTESIAN_POINT('',(0.012,0.00988380028027134,-0.00453369253696235));
#23979=CARTESIAN_POINT('Origin',(0.012,0.00707005305261661,-0.00817276199753401));
#23980=CARTESIAN_POINT('',(0.012,0.0100596045052361,-0.00412895061707364));
#23981=CARTESIAN_POINT('Origin',(0.012,0.,0.));
#23982=CARTESIAN_POINT('',(0.012,0.0112535852442972,-0.00416615159941835));
#23983=CARTESIAN_POINT('Origin',(0.012,0.0107986353290695,0.000411295349988523));
#23984=CARTESIAN_POINT('',(0.012,0.0113587411835337,-0.00387027114366614));
#23985=CARTESIAN_POINT('Origin',(0.012,0.,0.));
#23986=CARTESIAN_POINT('',(0.012,0.0104090797518856,-0.0031456215155173));
#23987=CARTESIAN_POINT('Origin',(0.012,0.00811705981202389,-0.00713393501814925));
#23988=CARTESIAN_POINT('',(0.012,0.010528134175832,-0.00272071071150138));
#23989=CARTESIAN_POINT('Origin',(0.012,0.,0.));
#23990=CARTESIAN_POINT('',(0.012,0.0117160596469668,-0.00259498484556562));
#23991=CARTESIAN_POINT('Origin',(0.012,0.0106420515472837,0.00187787851047546));
#23992=CARTESIAN_POINT('',(0.012,0.0117799471079179,-0.00228754150446667));
#23993=CARTESIAN_POINT('Origin',(0.012,0.,0.));
#23994=CARTESIAN_POINT('',(0.012,0.0107404577624574,-0.00169895351698263));
#23995=CARTESIAN_POINT('Origin',(0.012,0.00901286110520013,-0.00596221632729979));
#23996=CARTESIAN_POINT('',(0.012,0.0108005446267269,-0.0012617891131562));
#23997=CARTESIAN_POINT('Origin',(0.012,0.,0.));
#23998=CARTESIAN_POINT('',(0.012,0.0119602860260496,-0.000975478433939885));
#23999=CARTESIAN_POINT('Origin',(0.012,0.0102872264807069,0.00330948034739484));
#24000=CARTESIAN_POINT('',(0.012,0.0119817149061973,-0.000662199295233908));
#24001=CARTESIAN_POINT('Origin',(0.012,0.,0.));
#24002=CARTESIAN_POINT('',(0.012,0.0108717613666412,-0.000220637228970241));
#24003=CARTESIAN_POINT('Origin',(0.012,0.00974076984897452,-0.00467943282721939));
#24004=CARTESIAN_POINT('',(0.012,0.0108717613666412,0.000220637228970242));
#24005=CARTESIAN_POINT('Origin',(0.012,0.,0.));
#24006=CARTESIAN_POINT('',(0.012,0.0119817149061973,0.000662199295233908));
#24007=CARTESIAN_POINT('Origin',(0.012,0.00974076984897452,0.00467943282721939));
#24008=CARTESIAN_POINT('',(0.012,0.0119602860260496,0.00097547843394005));
#24009=CARTESIAN_POINT('Origin',(0.012,0.,0.));
#24010=CARTESIAN_POINT('',(0.012,0.0108005446267269,0.00126178911315635));
#24011=CARTESIAN_POINT('Origin',(0.012,0.0102872264807069,-0.00330948034739469));
#24012=CARTESIAN_POINT('',(0.012,0.0107404577624574,0.00169895351698278));
#24013=CARTESIAN_POINT('Origin',(0.012,0.,0.));
#24014=CARTESIAN_POINT('',(0.012,0.0117799471079178,0.00228754150446684));
#24015=CARTESIAN_POINT('Origin',(0.012,0.00901286110520005,0.00596221632729992));
#24016=CARTESIAN_POINT('',(0.012,0.0117160596469668,0.00259498484556578));
#24017=CARTESIAN_POINT('Origin',(0.012,0.,0.));
#24018=CARTESIAN_POINT('',(0.012,0.010528134175832,0.00272071071150152));
#24019=CARTESIAN_POINT('Origin',(0.012,0.0106420515472837,-0.00187787851047532));
#24020=CARTESIAN_POINT('',(0.012,0.0104090797518855,0.00314562151551744));
#24021=CARTESIAN_POINT('Origin',(0.012,0.,0.));
#24022=CARTESIAN_POINT('',(0.012,0.0113587411835337,0.0038702711436663));
#24023=CARTESIAN_POINT('Origin',(0.012,0.00811705981202379,0.00713393501814937));
#24024=CARTESIAN_POINT('',(0.012,0.0112535852442971,0.00416615159941851));
#24025=CARTESIAN_POINT('Origin',(0.012,0.,0.));
#24026=CARTESIAN_POINT('',(0.012,0.0100596045052361,0.00412895061707378));
#24027=CARTESIAN_POINT('Origin',(0.012,0.0107986353290695,-0.000411295349988374));
#24028=CARTESIAN_POINT('',(0.012,0.00988380028027128,0.00453369253696249));
#24029=CARTESIAN_POINT('Origin',(0.012,0.,0.));
#24030=CARTESIAN_POINT('',(0.012,0.0107259434024639,0.00538090495429348));
#24031=CARTESIAN_POINT('Origin',(0.012,0.0070700530526165,0.00817276199753411));
#24032=CARTESIAN_POINT('',(0.012,0.0105814778411272,0.00565971083163561));
#24033=CARTESIAN_POINT('Origin',(0.012,0.,0.));
#24034=CARTESIAN_POINT('',(0.012,0.00940368343621032,0.00546027598492453));
#24035=CARTESIAN_POINT('Origin',(0.012,0.0107540609664773,0.00106294946466816));
#24036=CARTESIAN_POINT('',(0.012,0.00917440431030386,0.00583730944451961));
#24037=CARTESIAN_POINT('Origin',(0.012,0.,0.));
#24038=CARTESIAN_POINT('',(0.012,0.0098933415900706,0.00679130268668532));
#24039=CARTESIAN_POINT('Origin',(0.012,0.00589134458189306,0.00905934588436432));
#24040=CARTESIAN_POINT('',(0.012,0.00971225752670205,0.00704784035964347));
#24041=CARTESIAN_POINT('Origin',(0.012,0.,0.));
#24042=CARTESIAN_POINT('',(0.012,0.00857258953722032,0.00668988674241506));
#24043=CARTESIAN_POINT('Origin',(0.012,0.0105091587955444,0.00251739354197556));
#24044=CARTESIAN_POINT('',(0.012,0.00829410654667506,0.00703218832173896));
#24045=CARTESIAN_POINT('Origin',(0.012,0.,0.));
#24046=CARTESIAN_POINT('',(0.012,0.00887644554277539,0.00807519129966237));
#24047=CARTESIAN_POINT('Origin',(0.012,0.00460289150846097,0.00977717129830952));
#24048=CARTESIAN_POINT('',(0.012,0.00866211623085135,0.00830468195677725));
#24049=CARTESIAN_POINT('Origin',(0.012,0.,0.));
#24050=CARTESIAN_POINT('',(0.012,0.00758180451511419,0.00779487756764621));
#24051=CARTESIAN_POINT('Origin',(0.012,0.0100684908803426,0.00392494334068744));
#24052=CARTESIAN_POINT('',(0.012,0.00725930527113395,0.00809607083593559));
#24053=CARTESIAN_POINT('Origin',(0.012,0.,0.));
#24054=CARTESIAN_POINT('',(0.012,0.00769419810989822,0.00920865437757541));
#24055=CARTESIAN_POINT('Origin',(0.012,0.00322869527523144,0.0103128665100857));
#24056=CARTESIAN_POINT('',(0.012,0.00745061609897321,0.00940682304211795));
#24057=CARTESIAN_POINT('Origin',(0.012,0.,0.));
#24058=CARTESIAN_POINT('',(0.012,0.00644978482021654,0.00875466457226685));
#24059=CARTESIAN_POINT('Origin',(0.012,0.00944026603035638,0.00525937887124031));
#24060=CARTESIAN_POINT('',(0.012,0.00608927687352466,0.00900913886881303));
#24061=CARTESIAN_POINT('Origin',(0.012,0.,0.));
#24062=CARTESIAN_POINT('',(0.012,0.00636862232421553,0.0101705776478774));
#24063=CARTESIAN_POINT('Origin',(0.012,0.00179435455795041,0.0106564525314718));
#24064=CARTESIAN_POINT('',(0.012,0.00610032508627822,0.0103337328125767));
#24065=CARTESIAN_POINT('Origin',(0.012,0.,0.));
#24066=CARTESIAN_POINT('',(0.012,0.00519761783757978,0.00955136874036766));
#24067=CARTESIAN_POINT('Origin',(0.012,0.00863618688589385,0.00649584212454895));
#24068=CARTESIAN_POINT('',(0.012,0.00480581676911591,0.00975438369050984));
#24069=CARTESIAN_POINT('Origin',(0.012,0.,0.));
#24070=CARTESIAN_POINT('',(0.012,0.00492441115452891,0.0109430423000714));
#24071=CARTESIAN_POINT('Origin',(0.012,0.00032658841030397,0.0108015290049791));
#24072=CARTESIAN_POINT('',(0.012,0.00463639655948419,0.0110681446929105));
#24073=CARTESIAN_POINT('Origin',(0.012,0.,0.));
#24074=CARTESIAN_POINT('',(0.012,0.00384862906889953,0.0101701489807191));
#24075=CARTESIAN_POINT('Origin',(0.012,0.00767123192004022,0.00761130012968254));
#24076=CARTESIAN_POINT('',(0.012,0.00343283339125305,0.0103179228000552));
#24077=CARTESIAN_POINT('Origin',(0.012,0.,0.));
#24078=CARTESIAN_POINT('',(0.012,0.00338846752237713,0.0115116587792462));
#24079=CARTESIAN_POINT('Origin',(0.012,-0.00114726146149743,0.0107453934304013));
#24080=CARTESIAN_POINT('',(0.012,0.00308610073718616,0.0115963779793494));
#24081=CARTESIAN_POINT('Origin',(0.012,0.,0.));
#24082=CARTESIAN_POINT('',(0.012,0.00242794762255152,0.0105994785882206));
#24083=CARTESIAN_POINT('Origin',(0.012,0.00656337641804445,0.00858497401453304));
#24084=CARTESIAN_POINT('',(0.012,0.00199590282248136,0.0106892585300951));
#24085=CARTESIAN_POINT('Origin',(0.012,0.,0.));
#24086=CARTESIAN_POINT('',(0.012,0.00178940315151022,0.0118658348362585));
#24087=CARTESIAN_POINT('Origin',(0.012,-0.00259974002297318,0.0104890915072804));
#24088=CARTESIAN_POINT('',(0.012,0.00147831669728117,0.0119085926852227));
#24089=CARTESIAN_POINT('Origin',(0.012,0.,0.));
#24090=CARTESIAN_POINT('',(0.012,0.000962038105848705,0.0108313599646072));
#24091=CARTESIAN_POINT('Origin',(0.012,0.00533325763176559,0.00939872607688742));
#24092=CARTESIAN_POINT('',(0.012,0.000521792360520001,0.0108614735985732));
#24093=CARTESIAN_POINT('Origin',(0.012,0.,0.));
#24094=CARTESIAN_POINT('',(0.012,0.000157005585611465,0.011998972841293));
#24095=CARTESIAN_POINT('Origin',(0.012,-0.00400379034671796,0.010037397655502));
#24096=CARTESIAN_POINT('Origin',(0.012,0.,0.));
#24097=CARTESIAN_POINT('',(0.012,-1.10218211923262E-18,-0.009));
#24098=CARTESIAN_POINT('Origin',(0.012,0.,0.));
#24099=CARTESIAN_POINT('Origin',(-0.01,0.,0.));
#24100=CARTESIAN_POINT('',(0.,-0.000157005585611549,0.011998972841293));
#24101=CARTESIAN_POINT('',(0.006,-0.000157005585611549,0.011998972841293));
#24102=CARTESIAN_POINT('',(0.,0.000157005585611465,0.011998972841293));
#24103=CARTESIAN_POINT('',(0.006,0.000157005585611465,0.011998972841293));
#24104=CARTESIAN_POINT('Origin',(0.,0.,0.));
#24105=CARTESIAN_POINT('Origin',(-0.01,0.,0.));
#24106=CARTESIAN_POINT('',(0.,-0.00147831669728126,0.0119085926852227));
#24107=CARTESIAN_POINT('',(0.006,-0.00147831669728126,0.0119085926852227));
#24108=CARTESIAN_POINT('',(0.,-0.0017894031515103,0.0118658348362585));
#24109=CARTESIAN_POINT('Origin',(0.,0.,0.));
#24110=CARTESIAN_POINT('',(0.006,-0.0017894031515103,0.0118658348362585));
#24111=CARTESIAN_POINT('Origin',(-0.01,0.,0.));
#24112=CARTESIAN_POINT('',(0.,0.00147831669728117,0.0119085926852227));
#24113=CARTESIAN_POINT('',(0.006,0.00147831669728117,0.0119085926852227));
#24114=CARTESIAN_POINT('',(0.,0.00178940315151022,0.0118658348362585));
#24115=CARTESIAN_POINT('',(0.006,0.00178940315151022,0.0118658348362585));
#24116=CARTESIAN_POINT('Origin',(0.,0.,0.));
#24117=CARTESIAN_POINT('Origin',(-0.01,0.,0.));
#24118=CARTESIAN_POINT('',(0.,0.00308610073718616,0.0115963779793494));
#24119=CARTESIAN_POINT('',(0.006,0.00308610073718616,0.0115963779793494));
#24120=CARTESIAN_POINT('',(0.,0.00338846752237713,0.0115116587792462));
#24121=CARTESIAN_POINT('',(0.006,0.00338846752237713,0.0115116587792462));
#24122=CARTESIAN_POINT('Origin',(0.,0.,0.));
#24123=CARTESIAN_POINT('Origin',(-0.01,0.,0.));
#24124=CARTESIAN_POINT('',(0.,0.00745061609897321,0.00940682304211795));
#24125=CARTESIAN_POINT('',(0.006,0.00745061609897321,0.00940682304211795));
#24126=CARTESIAN_POINT('',(0.,0.00769419810989822,0.00920865437757541));
#24127=CARTESIAN_POINT('',(0.006,0.00769419810989822,0.00920865437757541));
#24128=CARTESIAN_POINT('Origin',(0.,0.,0.));
#24129=CARTESIAN_POINT('Origin',(-0.01,0.,0.));
#24130=CARTESIAN_POINT('',(0.,0.00636862232421553,0.0101705776478774));
#24131=CARTESIAN_POINT('',(0.006,0.00636862232421553,0.0101705776478774));
#24132=CARTESIAN_POINT('',(0.,0.00610032508627822,0.0103337328125767));
#24133=CARTESIAN_POINT('Origin',(0.,0.,0.));
#24134=CARTESIAN_POINT('',(0.006,0.00610032508627822,0.0103337328125767));
#24135=CARTESIAN_POINT('Origin',(-0.01,0.,0.));
#24136=CARTESIAN_POINT('',(0.,0.00492441115452891,0.0109430423000714));
#24137=CARTESIAN_POINT('',(0.006,0.00492441115452891,0.0109430423000714));
#24138=CARTESIAN_POINT('',(0.,0.00463639655948419,0.0110681446929105));
#24139=CARTESIAN_POINT('Origin',(0.,0.,0.));
#24140=CARTESIAN_POINT('',(0.006,0.00463639655948419,0.0110681446929105));
#24141=CARTESIAN_POINT('Origin',(-0.01,0.,0.));
#24142=CARTESIAN_POINT('',(0.,0.0105814778411272,0.00565971083163561));
#24143=CARTESIAN_POINT('',(0.006,0.0105814778411272,0.00565971083163561));
#24144=CARTESIAN_POINT('',(0.,0.0107259434024639,0.00538090495429348));
#24145=CARTESIAN_POINT('',(0.006,0.0107259434024639,0.00538090495429348));
#24146=CARTESIAN_POINT('Origin',(0.,0.,0.));
#24147=CARTESIAN_POINT('Origin',(-0.01,0.,0.));
#24148=CARTESIAN_POINT('',(0.,0.0098933415900706,0.00679130268668532));
#24149=CARTESIAN_POINT('',(0.006,0.0098933415900706,0.00679130268668532));
#24150=CARTESIAN_POINT('',(0.,0.00971225752670205,0.00704784035964347));
#24151=CARTESIAN_POINT('Origin',(0.,0.,0.));
#24152=CARTESIAN_POINT('',(0.006,0.00971225752670205,0.00704784035964347));
#24153=CARTESIAN_POINT('Origin',(-0.01,0.,0.));
#24154=CARTESIAN_POINT('',(0.,0.00866211623085135,0.00830468195677725));
#24155=CARTESIAN_POINT('',(0.006,0.00866211623085135,0.00830468195677725));
#24156=CARTESIAN_POINT('',(0.,0.00887644554277539,0.00807519129966237));
#24157=CARTESIAN_POINT('',(0.006,0.00887644554277539,0.00807519129966237));
#24158=CARTESIAN_POINT('Origin',(0.,0.,0.));
#24159=CARTESIAN_POINT('Origin',(-0.01,0.,0.));
#24160=CARTESIAN_POINT('',(0.,0.0112535852442971,0.00416615159941851));
#24161=CARTESIAN_POINT('',(0.006,0.0112535852442971,0.00416615159941851));
#24162=CARTESIAN_POINT('',(0.,0.0113587411835337,0.0038702711436663));
#24163=CARTESIAN_POINT('',(0.006,0.0113587411835337,0.0038702711436663));
#24164=CARTESIAN_POINT('Origin',(0.,0.,0.));
#24165=CARTESIAN_POINT('Origin',(-0.01,0.,0.));
#24166=CARTESIAN_POINT('',(0.,0.0117160596469668,0.00259498484556578));
#24167=CARTESIAN_POINT('',(0.006,0.0117160596469668,0.00259498484556578));
#24168=CARTESIAN_POINT('',(0.,0.0117799471079178,0.00228754150446684));
#24169=CARTESIAN_POINT('',(0.006,0.0117799471079178,0.00228754150446684));
#24170=CARTESIAN_POINT('Origin',(0.,0.,0.));
#24171=CARTESIAN_POINT('Origin',(-0.01,0.,0.));
#24172=CARTESIAN_POINT('',(0.,-0.0119817149061973,0.000662199295233824));
#24173=CARTESIAN_POINT('',(0.006,-0.0119817149061973,0.000662199295233823));
#24174=CARTESIAN_POINT('',(0.,-0.0119602860260496,0.000975478433939967));
#24175=CARTESIAN_POINT('',(0.006,-0.0119602860260496,0.000975478433939967));
#24176=CARTESIAN_POINT('Origin',(0.,0.,0.));
#24177=CARTESIAN_POINT('Origin',(-0.01,0.,0.));
#24178=CARTESIAN_POINT('',(0.,-0.0119817149061973,-0.000662199295233991));
#24179=CARTESIAN_POINT('',(0.006,-0.0119817149061973,-0.000662199295233991));
#24180=CARTESIAN_POINT('',(0.,-0.0119602860260496,-0.000975478433940136));
#24181=CARTESIAN_POINT('Origin',(0.,0.,0.));
#24182=CARTESIAN_POINT('',(0.006,-0.0119602860260496,-0.000975478433940136));
#24183=CARTESIAN_POINT('Origin',(-0.01,0.,0.));
#24184=CARTESIAN_POINT('',(0.,-0.0117799471079178,0.00228754150446675));
#24185=CARTESIAN_POINT('',(0.006,-0.0117799471079178,0.00228754150446675));
#24186=CARTESIAN_POINT('',(0.,-0.0117160596469668,0.0025949848455657));
#24187=CARTESIAN_POINT('',(0.006,-0.0117160596469668,0.0025949848455657));
#24188=CARTESIAN_POINT('Origin',(0.,0.,0.));
#24189=CARTESIAN_POINT('Origin',(-0.01,0.,0.));
#24190=CARTESIAN_POINT('',(0.,-0.0113587411835337,0.00387027114366622));
#24191=CARTESIAN_POINT('',(0.006,-0.0113587411835337,0.00387027114366622));
#24192=CARTESIAN_POINT('',(0.,-0.0112535852442972,0.00416615159941843));
#24193=CARTESIAN_POINT('',(0.006,-0.0112535852442972,0.00416615159941843));
#24194=CARTESIAN_POINT('Origin',(0.,0.,0.));
#24195=CARTESIAN_POINT('Origin',(-0.01,0.,0.));
#24196=CARTESIAN_POINT('',(0.,-0.00887644554277545,0.00807519129966231));
#24197=CARTESIAN_POINT('',(0.006,-0.00887644554277545,0.00807519129966231));
#24198=CARTESIAN_POINT('',(0.,-0.00866211623085141,0.00830468195677719));
#24199=CARTESIAN_POINT('',(0.006,-0.00866211623085141,0.00830468195677719));
#24200=CARTESIAN_POINT('Origin',(0.,0.,0.));
#24201=CARTESIAN_POINT('Origin',(-0.01,0.,0.));
#24202=CARTESIAN_POINT('',(0.,-0.0097122575267021,0.0070478403596434));
#24203=CARTESIAN_POINT('',(0.006,-0.0097122575267021,0.0070478403596434));
#24204=CARTESIAN_POINT('',(0.,-0.00989334159007065,0.00679130268668526));
#24205=CARTESIAN_POINT('Origin',(0.,0.,0.));
#24206=CARTESIAN_POINT('',(0.006,-0.00989334159007065,0.00679130268668526));
#24207=CARTESIAN_POINT('Origin',(-0.01,0.,0.));
#24208=CARTESIAN_POINT('',(0.,-0.0105814778411273,0.00565971083163554));
#24209=CARTESIAN_POINT('',(0.006,-0.0105814778411273,0.00565971083163554));
#24210=CARTESIAN_POINT('',(0.,-0.010725943402464,0.0053809049542934));
#24211=CARTESIAN_POINT('Origin',(0.,0.,0.));
#24212=CARTESIAN_POINT('',(0.006,-0.010725943402464,0.0053809049542934));
#24213=CARTESIAN_POINT('Origin',(-0.01,0.,0.));
#24214=CARTESIAN_POINT('',(0.,-0.00492441115452898,0.0109430423000713));
#24215=CARTESIAN_POINT('',(0.006,-0.00492441115452898,0.0109430423000713));
#24216=CARTESIAN_POINT('',(0.,-0.00463639655948427,0.0110681446929105));
#24217=CARTESIAN_POINT('',(0.006,-0.00463639655948427,0.0110681446929105));
#24218=CARTESIAN_POINT('Origin',(0.,0.,0.));
#24219=CARTESIAN_POINT('Origin',(-0.01,0.,0.));
#24220=CARTESIAN_POINT('',(0.,-0.00610032508627829,0.0103337328125767));
#24221=CARTESIAN_POINT('',(0.006,-0.00610032508627829,0.0103337328125767));
#24222=CARTESIAN_POINT('',(0.,-0.0063686223242156,0.0101705776478774));
#24223=CARTESIAN_POINT('Origin',(0.,0.,0.));
#24224=CARTESIAN_POINT('',(0.006,-0.0063686223242156,0.0101705776478774));
#24225=CARTESIAN_POINT('Origin',(-0.01,0.,0.));
#24226=CARTESIAN_POINT('',(0.,-0.00769419810989828,0.00920865437757535));
#24227=CARTESIAN_POINT('',(0.006,-0.00769419810989828,0.00920865437757535));
#24228=CARTESIAN_POINT('',(0.,-0.00745061609897327,0.0094068230421179));
#24229=CARTESIAN_POINT('',(0.006,-0.00745061609897327,0.0094068230421179));
#24230=CARTESIAN_POINT('Origin',(0.,0.,0.));
#24231=CARTESIAN_POINT('Origin',(-0.01,0.,0.));
#24232=CARTESIAN_POINT('',(0.,-0.00338846752237721,0.0115116587792461));
#24233=CARTESIAN_POINT('',(0.006,-0.00338846752237721,0.0115116587792461));
#24234=CARTESIAN_POINT('',(0.,-0.00308610073718624,0.0115963779793493));
#24235=CARTESIAN_POINT('',(0.006,-0.00308610073718624,0.0115963779793493));
#24236=CARTESIAN_POINT('Origin',(0.,0.,0.));
#24237=CARTESIAN_POINT('Origin',(-0.01,0.,0.));
#24238=CARTESIAN_POINT('',(0.,-0.00147831669728109,-0.0119085926852227));
#24239=CARTESIAN_POINT('',(0.006,-0.00147831669728109,-0.0119085926852227));
#24240=CARTESIAN_POINT('',(0.,-0.00178940315151014,-0.0118658348362585));
#24241=CARTESIAN_POINT('',(0.006,-0.00178940315151014,-0.0118658348362585));
#24242=CARTESIAN_POINT('Origin',(0.,0.,0.));
#24243=CARTESIAN_POINT('Origin',(-0.01,0.,0.));
#24244=CARTESIAN_POINT('',(0.,-0.000157005585611382,-0.011998972841293));
#24245=CARTESIAN_POINT('',(0.006,-0.000157005585611383,-0.011998972841293));
#24246=CARTESIAN_POINT('',(0.,0.000157005585611632,-0.011998972841293));
#24247=CARTESIAN_POINT('Origin',(0.,0.,0.));
#24248=CARTESIAN_POINT('',(0.006,0.000157005585611632,-0.011998972841293));
#24249=CARTESIAN_POINT('Origin',(-0.01,0.,0.));
#24250=CARTESIAN_POINT('',(0.,-0.00308610073718608,-0.0115963779793494));
#24251=CARTESIAN_POINT('',(0.006,-0.00308610073718608,-0.0115963779793494));
#24252=CARTESIAN_POINT('',(0.,-0.00338846752237705,-0.0115116587792462));
#24253=CARTESIAN_POINT('',(0.006,-0.00338846752237705,-0.0115116587792462));
#24254=CARTESIAN_POINT('Origin',(0.,0.,0.));
#24255=CARTESIAN_POINT('Origin',(-0.01,0.,0.));
#24256=CARTESIAN_POINT('',(0.,-0.00463639655948412,-0.0110681446929105));
#24257=CARTESIAN_POINT('',(0.006,-0.00463639655948412,-0.0110681446929105));
#24258=CARTESIAN_POINT('',(0.,-0.00492441115452883,-0.0109430423000714));
#24259=CARTESIAN_POINT('',(0.006,-0.00492441115452883,-0.0109430423000714));
#24260=CARTESIAN_POINT('Origin',(0.,0.,0.));
#24261=CARTESIAN_POINT('Origin',(-0.01,0.,0.));
#24262=CARTESIAN_POINT('',(0.,-0.00866211623085129,-0.00830468195677731));
#24263=CARTESIAN_POINT('',(0.006,-0.00866211623085129,-0.0083046819567773));
#24264=CARTESIAN_POINT('',(0.,-0.00887644554277534,-0.00807519129966243));
#24265=CARTESIAN_POINT('',(0.006,-0.00887644554277533,-0.00807519129966243));
#24266=CARTESIAN_POINT('Origin',(0.,0.,0.));
#24267=CARTESIAN_POINT('Origin',(-0.01,0.,0.));
#24268=CARTESIAN_POINT('',(0.,-0.00769419810989815,-0.00920865437757546));
#24269=CARTESIAN_POINT('',(0.006,-0.00769419810989815,-0.00920865437757546));
#24270=CARTESIAN_POINT('',(0.,-0.00745061609897314,-0.009406823042118));
#24271=CARTESIAN_POINT('Origin',(0.,0.,0.));
#24272=CARTESIAN_POINT('',(0.006,-0.00745061609897314,-0.009406823042118));
#24273=CARTESIAN_POINT('Origin',(-0.01,0.,0.));
#24274=CARTESIAN_POINT('',(0.,-0.00610032508627815,-0.0103337328125767));
#24275=CARTESIAN_POINT('',(0.006,-0.00610032508627815,-0.0103337328125767));
#24276=CARTESIAN_POINT('',(0.,-0.00636862232421547,-0.0101705776478774));
#24277=CARTESIAN_POINT('',(0.006,-0.00636862232421547,-0.0101705776478774));
#24278=CARTESIAN_POINT('Origin',(0.,0.,0.));
#24279=CARTESIAN_POINT('Origin',(-0.01,0.,0.));
#24280=CARTESIAN_POINT('',(0.,-0.0105814778411272,-0.00565971083163568));
#24281=CARTESIAN_POINT('',(0.006,-0.0105814778411272,-0.00565971083163568));
#24282=CARTESIAN_POINT('',(0.,-0.0107259434024639,-0.00538090495429355));
#24283=CARTESIAN_POINT('',(0.006,-0.0107259434024639,-0.00538090495429355));
#24284=CARTESIAN_POINT('Origin',(0.,0.,0.));
#24285=CARTESIAN_POINT('Origin',(-0.01,0.,0.));
#24286=CARTESIAN_POINT('',(0.,-0.00989334159007055,-0.00679130268668539));
#24287=CARTESIAN_POINT('',(0.006,-0.00989334159007055,-0.00679130268668539));
#24288=CARTESIAN_POINT('',(0.,-0.009712257526702,-0.00704784035964354));
#24289=CARTESIAN_POINT('Origin',(0.,0.,0.));
#24290=CARTESIAN_POINT('',(0.006,-0.009712257526702,-0.00704784035964354));
#24291=CARTESIAN_POINT('Origin',(-0.01,0.,0.));
#24292=CARTESIAN_POINT('',(0.,-0.0112535852442971,-0.00416615159941858));
#24293=CARTESIAN_POINT('',(0.006,-0.0112535852442971,-0.00416615159941858));
#24294=CARTESIAN_POINT('',(0.,-0.0113587411835336,-0.00387027114366637));
#24295=CARTESIAN_POINT('',(0.006,-0.0113587411835336,-0.00387027114366637));
#24296=CARTESIAN_POINT('Origin',(0.,0.,0.));
#24297=CARTESIAN_POINT('Origin',(-0.01,0.,0.));
#24298=CARTESIAN_POINT('',(0.,-0.0117160596469668,-0.00259498484556586));
#24299=CARTESIAN_POINT('',(0.006,-0.0117160596469668,-0.00259498484556586));
#24300=CARTESIAN_POINT('',(0.,-0.0117799471079178,-0.00228754150446692));
#24301=CARTESIAN_POINT('',(0.006,-0.0117799471079178,-0.00228754150446692));
#24302=CARTESIAN_POINT('Origin',(0.,0.,0.));
#24303=CARTESIAN_POINT('Origin',(-0.01,0.,0.));
#24304=CARTESIAN_POINT('',(0.,0.0117799471079179,-0.00228754150446667));
#24305=CARTESIAN_POINT('',(0.006,0.0117799471079179,-0.00228754150446667));
#24306=CARTESIAN_POINT('',(0.,0.0117160596469668,-0.00259498484556562));
#24307=CARTESIAN_POINT('',(0.006,0.0117160596469668,-0.00259498484556562));
#24308=CARTESIAN_POINT('Origin',(0.,0.,0.));
#24309=CARTESIAN_POINT('Origin',(-0.01,0.,0.));
#24310=CARTESIAN_POINT('',(0.,0.0119602860260496,-0.000975478433939885));
#24311=CARTESIAN_POINT('',(0.006,0.0119602860260496,-0.000975478433939885));
#24312=CARTESIAN_POINT('',(0.,0.0119817149061973,-0.000662199295233908));
#24313=CARTESIAN_POINT('Origin',(0.,0.,0.));
#24314=CARTESIAN_POINT('',(0.006,0.0119817149061973,-0.000662199295233907));
#24315=CARTESIAN_POINT('Origin',(-0.01,0.,0.));
#24316=CARTESIAN_POINT('',(0.,0.0113587411835337,-0.00387027114366614));
#24317=CARTESIAN_POINT('',(0.006,0.0113587411835337,-0.00387027114366614));
#24318=CARTESIAN_POINT('',(0.,0.0112535852442972,-0.00416615159941835));
#24319=CARTESIAN_POINT('',(0.006,0.0112535852442972,-0.00416615159941835));
#24320=CARTESIAN_POINT('Origin',(0.,0.,0.));
#24321=CARTESIAN_POINT('Origin',(-0.01,0.,0.));
#24322=CARTESIAN_POINT('',(0.,0.010725943402464,-0.00538090495429333));
#24323=CARTESIAN_POINT('',(0.006,0.010725943402464,-0.00538090495429333));
#24324=CARTESIAN_POINT('',(0.,0.0105814778411273,-0.00565971083163546));
#24325=CARTESIAN_POINT('',(0.006,0.0105814778411273,-0.00565971083163546));
#24326=CARTESIAN_POINT('Origin',(0.,0.,0.));
#24327=CARTESIAN_POINT('Origin',(-0.01,0.,0.));
#24328=CARTESIAN_POINT('',(0.,0.00769419810989834,-0.0092086543775753));
#24329=CARTESIAN_POINT('',(0.006,0.00769419810989834,-0.0092086543775753));
#24330=CARTESIAN_POINT('',(0.,0.00745061609897333,-0.00940682304211785));
#24331=CARTESIAN_POINT('',(0.006,0.00745061609897333,-0.00940682304211785));
#24332=CARTESIAN_POINT('Origin',(0.,0.,0.));
#24333=CARTESIAN_POINT('Origin',(-0.01,0.,0.));
#24334=CARTESIAN_POINT('',(0.,0.00866211623085146,-0.00830468195677713));
#24335=CARTESIAN_POINT('',(0.006,0.00866211623085146,-0.00830468195677713));
#24336=CARTESIAN_POINT('',(0.,0.0088764455427755,-0.00807519129966225));
#24337=CARTESIAN_POINT('Origin',(0.,0.,0.));
#24338=CARTESIAN_POINT('',(0.006,0.0088764455427755,-0.00807519129966225));
#24339=CARTESIAN_POINT('Origin',(-0.01,0.,0.));
#24340=CARTESIAN_POINT('',(0.,0.00989334159007069,-0.00679130268668519));
#24341=CARTESIAN_POINT('',(0.006,0.00989334159007069,-0.00679130268668519));
#24342=CARTESIAN_POINT('',(0.,0.00971225752670214,-0.00704784035964334));
#24343=CARTESIAN_POINT('',(0.006,0.00971225752670214,-0.00704784035964334));
#24344=CARTESIAN_POINT('Origin',(0.,0.,0.));
#24345=CARTESIAN_POINT('Origin',(-0.01,0.,0.));
#24346=CARTESIAN_POINT('',(0.,0.00492441115452905,-0.0109430423000713));
#24347=CARTESIAN_POINT('',(0.006,0.00492441115452905,-0.0109430423000713));
#24348=CARTESIAN_POINT('',(0.,0.00463639655948435,-0.0110681446929104));
#24349=CARTESIAN_POINT('',(0.006,0.00463639655948435,-0.0110681446929104));
#24350=CARTESIAN_POINT('Origin',(0.,0.,0.));
#24351=CARTESIAN_POINT('Origin',(-0.01,0.,0.));
#24352=CARTESIAN_POINT('',(0.,0.00610032508627836,-0.0103337328125766));
#24353=CARTESIAN_POINT('',(0.006,0.00610032508627836,-0.0103337328125766));
#24354=CARTESIAN_POINT('',(0.,0.00636862232421567,-0.0101705776478773));
#24355=CARTESIAN_POINT('Origin',(0.,0.,0.));
#24356=CARTESIAN_POINT('',(0.006,0.00636862232421567,-0.0101705776478773));
#24357=CARTESIAN_POINT('Origin',(-0.01,0.,0.));
#24358=CARTESIAN_POINT('',(0.,0.00338846752237729,-0.0115116587792461));
#24359=CARTESIAN_POINT('',(0.006,0.00338846752237729,-0.0115116587792461));
#24360=CARTESIAN_POINT('',(0.,0.00308610073718632,-0.0115963779793493));
#24361=CARTESIAN_POINT('',(0.006,0.00308610073718632,-0.0115963779793493));
#24362=CARTESIAN_POINT('Origin',(0.,0.,0.));
#24363=CARTESIAN_POINT('Origin',(-0.01,0.,0.));
#24364=CARTESIAN_POINT('',(0.,0.00178940315151039,-0.0118658348362584));
#24365=CARTESIAN_POINT('',(0.006,0.00178940315151039,-0.0118658348362584));
#24366=CARTESIAN_POINT('',(0.,0.00147831669728134,-0.0119085926852227));
#24367=CARTESIAN_POINT('',(0.006,0.00147831669728134,-0.0119085926852227));
#24368=CARTESIAN_POINT('Origin',(0.,0.,0.));
#24369=CARTESIAN_POINT('Origin',(0.,0.,0.));
#24370=CARTESIAN_POINT('',(0.,-0.000521792360520078,0.0108614735985732));
#24371=CARTESIAN_POINT('Origin',(0.,0.00400379034671789,0.010037397655502));
#24372=CARTESIAN_POINT('',(0.,0.000521792360520001,0.0108614735985732));
#24373=CARTESIAN_POINT('Origin',(0.,-0.00400379034671796,0.010037397655502));
#24374=CARTESIAN_POINT('',(0.,0.000962038105848705,0.0108313599646072));
#24375=CARTESIAN_POINT('Origin',(0.,0.,0.));
#24376=CARTESIAN_POINT('Origin',(0.,0.00533325763176559,0.00939872607688742));
#24377=CARTESIAN_POINT('',(0.,0.00199590282248136,0.0106892585300951));
#24378=CARTESIAN_POINT('Origin',(0.,-0.00259974002297318,0.0104890915072804));
#24379=CARTESIAN_POINT('',(0.,0.00242794762255152,0.0105994785882206));
#24380=CARTESIAN_POINT('Origin',(0.,0.,0.));
#24381=CARTESIAN_POINT('Origin',(0.,0.00656337641804445,0.00858497401453304));
#24382=CARTESIAN_POINT('',(0.,0.00343283339125305,0.0103179228000552));
#24383=CARTESIAN_POINT('Origin',(0.,-0.00114726146149743,0.0107453934304013));
#24384=CARTESIAN_POINT('',(0.,0.00384862906889953,0.0101701489807191));
#24385=CARTESIAN_POINT('Origin',(0.,0.,0.));
#24386=CARTESIAN_POINT('Origin',(0.,0.00767123192004022,0.00761130012968254));
#24387=CARTESIAN_POINT('',(0.,0.00480581676911591,0.00975438369050984));
#24388=CARTESIAN_POINT('Origin',(0.,0.00032658841030397,0.0108015290049791));
#24389=CARTESIAN_POINT('',(0.,0.00519761783757978,0.00955136874036766));
#24390=CARTESIAN_POINT('Origin',(0.,0.,0.));
#24391=CARTESIAN_POINT('Origin',(0.,0.00863618688589385,0.00649584212454895));
#24392=CARTESIAN_POINT('',(0.,0.00608927687352466,0.00900913886881303));
#24393=CARTESIAN_POINT('Origin',(0.,0.00179435455795041,0.0106564525314718));
#24394=CARTESIAN_POINT('',(0.,0.00644978482021654,0.00875466457226685));
#24395=CARTESIAN_POINT('Origin',(0.,0.,0.));
#24396=CARTESIAN_POINT('Origin',(0.,0.00944026603035638,0.00525937887124031));
#24397=CARTESIAN_POINT('',(0.,0.00725930527113395,0.00809607083593559));
#24398=CARTESIAN_POINT('Origin',(0.,0.00322869527523144,0.0103128665100857));
#24399=CARTESIAN_POINT('',(0.,0.00758180451511419,0.00779487756764621));
#24400=CARTESIAN_POINT('Origin',(0.,0.,0.));
#24401=CARTESIAN_POINT('Origin',(0.,0.0100684908803426,0.00392494334068744));
#24402=CARTESIAN_POINT('',(0.,0.00829410654667506,0.00703218832173896));
#24403=CARTESIAN_POINT('Origin',(0.,0.00460289150846097,0.00977717129830952));
#24404=CARTESIAN_POINT('',(0.,0.00857258953722032,0.00668988674241506));
#24405=CARTESIAN_POINT('Origin',(0.,0.,0.));
#24406=CARTESIAN_POINT('Origin',(0.,0.0105091587955444,0.00251739354197556));
#24407=CARTESIAN_POINT('',(0.,0.00917440431030386,0.00583730944451961));
#24408=CARTESIAN_POINT('Origin',(0.,0.00589134458189306,0.00905934588436432));
#24409=CARTESIAN_POINT('',(0.,0.00940368343621032,0.00546027598492453));
#24410=CARTESIAN_POINT('Origin',(0.,0.,0.));
#24411=CARTESIAN_POINT('Origin',(0.,0.0107540609664773,0.00106294946466816));
#24412=CARTESIAN_POINT('',(0.,0.00988380028027128,0.00453369253696249));
#24413=CARTESIAN_POINT('Origin',(0.,0.0070700530526165,0.00817276199753411));
#24414=CARTESIAN_POINT('',(0.,0.0100596045052361,0.00412895061707378));
#24415=CARTESIAN_POINT('Origin',(0.,0.,0.));
#24416=CARTESIAN_POINT('Origin',(0.,0.0107986353290695,-0.000411295349988374));
#24417=CARTESIAN_POINT('',(0.,0.0104090797518855,0.00314562151551744));
#24418=CARTESIAN_POINT('Origin',(0.,0.00811705981202379,0.00713393501814937));
#24419=CARTESIAN_POINT('',(0.,0.010528134175832,0.00272071071150152));
#24420=CARTESIAN_POINT('Origin',(0.,0.,0.));
#24421=CARTESIAN_POINT('Origin',(0.,0.0106420515472837,-0.00187787851047532));
#24422=CARTESIAN_POINT('',(0.,0.0107404577624574,0.00169895351698278));
#24423=CARTESIAN_POINT('Origin',(0.,0.00901286110520005,0.00596221632729992));
#24424=CARTESIAN_POINT('',(0.,0.0108005446267269,0.00126178911315635));
#24425=CARTESIAN_POINT('Origin',(0.,0.,0.));
#24426=CARTESIAN_POINT('',(0.,0.0119602860260496,0.00097547843394005));
#24427=CARTESIAN_POINT('Origin',(0.,0.0102872264807069,-0.00330948034739469));
#24428=CARTESIAN_POINT('',(0.,0.0119817149061973,0.000662199295233908));
#24429=CARTESIAN_POINT('Origin',(0.,0.,0.));
#24430=CARTESIAN_POINT('',(0.,0.0108717613666412,0.000220637228970242));
#24431=CARTESIAN_POINT('Origin',(0.,0.00974076984897452,0.00467943282721939));
#24432=CARTESIAN_POINT('',(0.,0.0108717613666412,-0.000220637228970241));
#24433=CARTESIAN_POINT('Origin',(0.,0.,0.));
#24434=CARTESIAN_POINT('Origin',(0.,0.00974076984897452,-0.00467943282721939));
#24435=CARTESIAN_POINT('',(0.,0.0108005446267269,-0.0012617891131562));
#24436=CARTESIAN_POINT('Origin',(0.,0.0102872264807069,0.00330948034739484));
#24437=CARTESIAN_POINT('',(0.,0.0107404577624574,-0.00169895351698263));
#24438=CARTESIAN_POINT('Origin',(0.,0.,0.));
#24439=CARTESIAN_POINT('Origin',(0.,0.00901286110520013,-0.00596221632729979));
#24440=CARTESIAN_POINT('',(0.,0.010528134175832,-0.00272071071150138));
#24441=CARTESIAN_POINT('Origin',(0.,0.0106420515472837,0.00187787851047546));
#24442=CARTESIAN_POINT('',(0.,0.0104090797518856,-0.0031456215155173));
#24443=CARTESIAN_POINT('Origin',(0.,0.,0.));
#24444=CARTESIAN_POINT('Origin',(0.,0.00811705981202389,-0.00713393501814925));
#24445=CARTESIAN_POINT('',(0.,0.0100596045052361,-0.00412895061707364));
#24446=CARTESIAN_POINT('Origin',(0.,0.0107986353290695,0.000411295349988523));
#24447=CARTESIAN_POINT('',(0.,0.00988380028027134,-0.00453369253696235));
#24448=CARTESIAN_POINT('Origin',(0.,0.,0.));
#24449=CARTESIAN_POINT('Origin',(0.,0.00707005305261661,-0.00817276199753401));
#24450=CARTESIAN_POINT('',(0.,0.0094036834362104,-0.0054602759849244));
#24451=CARTESIAN_POINT('Origin',(0.,0.0107540609664773,-0.00106294946466802));
#24452=CARTESIAN_POINT('',(0.,0.00917440431030394,-0.00583730944451949));
#24453=CARTESIAN_POINT('Origin',(0.,0.,0.));
#24454=CARTESIAN_POINT('Origin',(0.,0.00589134458189318,-0.00905934588436424));
#24455=CARTESIAN_POINT('',(0.,0.00857258953722041,-0.00668988674241494));
#24456=CARTESIAN_POINT('Origin',(0.,0.0105091587955445,-0.00251739354197541));
#24457=CARTESIAN_POINT('',(0.,0.00829410654667516,-0.00703218832173885));
#24458=CARTESIAN_POINT('Origin',(0.,0.,0.));
#24459=CARTESIAN_POINT('Origin',(0.,0.0046028915084611,-0.00977717129830945));
#24460=CARTESIAN_POINT('',(0.,0.0075818045151143,-0.0077948775676461));
#24461=CARTESIAN_POINT('Origin',(0.,0.0100684908803427,-0.0039249433406873));
#24462=CARTESIAN_POINT('',(0.,0.00725930527113406,-0.00809607083593549));
#24463=CARTESIAN_POINT('Origin',(0.,0.,0.));
#24464=CARTESIAN_POINT('Origin',(0.,0.00322869527523158,-0.0103128665100857));
#24465=CARTESIAN_POINT('',(0.,0.00644978482021666,-0.00875466457226676));
#24466=CARTESIAN_POINT('Origin',(0.,0.00944026603035645,-0.00525937887124018));
#24467=CARTESIAN_POINT('',(0.,0.00608927687352479,-0.00900913886881295));
#24468=CARTESIAN_POINT('Origin',(0.,0.,0.));
#24469=CARTESIAN_POINT('Origin',(0.,0.00179435455795055,-0.0106564525314718));
#24470=CARTESIAN_POINT('',(0.,0.00519761783757991,-0.00955136874036759));
#24471=CARTESIAN_POINT('Origin',(0.,0.00863618688589394,-0.00649584212454884));
#24472=CARTESIAN_POINT('',(0.,0.00480581676911604,-0.00975438369050977));
#24473=CARTESIAN_POINT('Origin',(0.,0.,0.));
#24474=CARTESIAN_POINT('Origin',(0.,0.000326588410304114,-0.0108015290049791));
#24475=CARTESIAN_POINT('',(0.,0.00384862906889967,-0.010170148980719));
#24476=CARTESIAN_POINT('Origin',(0.,0.00767123192004033,-0.00761130012968243));
#24477=CARTESIAN_POINT('',(0.,0.00343283339125319,-0.0103179228000551));
#24478=CARTESIAN_POINT('Origin',(0.,0.,0.));
#24479=CARTESIAN_POINT('Origin',(0.,-0.00114726146149728,-0.0107453934304014));
#24480=CARTESIAN_POINT('',(0.,0.00242794762255167,-0.0105994785882205));
#24481=CARTESIAN_POINT('Origin',(0.,0.00656337641804457,-0.00858497401453295));
#24482=CARTESIAN_POINT('',(0.,0.00199590282248151,-0.0106892585300951));
#24483=CARTESIAN_POINT('Origin',(0.,0.,0.));
#24484=CARTESIAN_POINT('Origin',(0.,-0.00259974002297304,-0.0104890915072804));
#24485=CARTESIAN_POINT('',(0.,0.000962038105848858,-0.0108313599646072));
#24486=CARTESIAN_POINT('Origin',(0.,0.00533325763176572,-0.00939872607688735));
#24487=CARTESIAN_POINT('',(0.,0.000521792360520154,-0.0108614735985732));
#24488=CARTESIAN_POINT('Origin',(0.,0.,0.));
#24489=CARTESIAN_POINT('Origin',(0.,-0.00400379034671782,-0.0100373976555021));
#24490=CARTESIAN_POINT('',(0.,-0.000521792360519925,-0.0108614735985732));
#24491=CARTESIAN_POINT('Origin',(0.,0.00400379034671803,-0.010037397655502));
#24492=CARTESIAN_POINT('',(0.,-0.00096203810584863,-0.0108313599646072));
#24493=CARTESIAN_POINT('Origin',(0.,0.,0.));
#24494=CARTESIAN_POINT('Origin',(0.,-0.00533325763176552,-0.00939872607688746));
#24495=CARTESIAN_POINT('',(0.,-0.00199590282248128,-0.0106892585300951));
#24496=CARTESIAN_POINT('Origin',(0.,0.00259974002297325,-0.0104890915072803));
#24497=CARTESIAN_POINT('',(0.,-0.00242794762255145,-0.0105994785882206));
#24498=CARTESIAN_POINT('Origin',(0.,0.,0.));
#24499=CARTESIAN_POINT('Origin',(0.,-0.00656337641804439,-0.00858497401453309));
#24500=CARTESIAN_POINT('',(0.,-0.00343283339125298,-0.0103179228000552));
#24501=CARTESIAN_POINT('Origin',(0.,0.0011472614614975,-0.0107453934304013));
#24502=CARTESIAN_POINT('',(0.,-0.00384862906889946,-0.0101701489807191));
#24503=CARTESIAN_POINT('Origin',(0.,0.,0.));
#24504=CARTESIAN_POINT('Origin',(0.,-0.00767123192004017,-0.00761130012968259));
#24505=CARTESIAN_POINT('',(0.,-0.00480581676911584,-0.00975438369050987));
#24506=CARTESIAN_POINT('Origin',(0.,-0.000326588410303897,-0.0108015290049791));
#24507=CARTESIAN_POINT('',(0.,-0.00519761783757972,-0.00955136874036769));
#24508=CARTESIAN_POINT('Origin',(0.,0.,0.));
#24509=CARTESIAN_POINT('Origin',(0.,-0.00863618688589381,-0.00649584212454901));
#24510=CARTESIAN_POINT('',(0.,-0.0060892768735246,-0.00900913886881307));
#24511=CARTESIAN_POINT('Origin',(0.,-0.00179435455795034,-0.0106564525314718));
#24512=CARTESIAN_POINT('',(0.,-0.00644978482021648,-0.00875466457226689));
#24513=CARTESIAN_POINT('Origin',(0.,0.,0.));
#24514=CARTESIAN_POINT('Origin',(0.,-0.00944026603035634,-0.00525937887124037));
#24515=CARTESIAN_POINT('',(0.,-0.0072593052711339,-0.00809607083593564));
#24516=CARTESIAN_POINT('Origin',(0.,-0.00322869527523136,-0.0103128665100857));
#24517=CARTESIAN_POINT('',(0.,-0.00758180451511414,-0.00779487756764626));
#24518=CARTESIAN_POINT('Origin',(0.,0.,0.));
#24519=CARTESIAN_POINT('Origin',(0.,-0.0100684908803426,-0.00392494334068751));
#24520=CARTESIAN_POINT('',(0.,-0.00829410654667501,-0.00703218832173902));
#24521=CARTESIAN_POINT('Origin',(0.,-0.0046028915084609,-0.00977717129830955));
#24522=CARTESIAN_POINT('',(0.,-0.00857258953722027,-0.00668988674241512));
#24523=CARTESIAN_POINT('Origin',(0.,0.,0.));
#24524=CARTESIAN_POINT('Origin',(0.,-0.0105091587955444,-0.00251739354197563));
#24525=CARTESIAN_POINT('',(0.,-0.00917440431030382,-0.00583730944451968));
#24526=CARTESIAN_POINT('Origin',(0.,-0.00589134458189299,-0.00905934588436437));
#24527=CARTESIAN_POINT('',(0.,-0.00940368343621029,-0.0054602759849246));
#24528=CARTESIAN_POINT('Origin',(0.,0.,0.));
#24529=CARTESIAN_POINT('Origin',(0.,-0.0107540609664773,-0.00106294946466824));
#24530=CARTESIAN_POINT('',(0.,-0.00988380028027125,-0.00453369253696255));
#24531=CARTESIAN_POINT('Origin',(0.,-0.00707005305261645,-0.00817276199753415));
#24532=CARTESIAN_POINT('',(0.,-0.010059604505236,-0.00412895061707385));
#24533=CARTESIAN_POINT('Origin',(0.,0.,0.));
#24534=CARTESIAN_POINT('Origin',(0.,-0.0107986353290695,0.0004112953499883));
#24535=CARTESIAN_POINT('',(0.,-0.0104090797518855,-0.00314562151551751));
#24536=CARTESIAN_POINT('Origin',(0.,-0.00811705981202375,-0.00713393501814942));
#24537=CARTESIAN_POINT('',(0.,-0.0105281341758319,-0.00272071071150159));
#24538=CARTESIAN_POINT('Origin',(0.,0.,0.));
#24539=CARTESIAN_POINT('Origin',(0.,-0.0106420515472838,0.00187787851047525));
#24540=CARTESIAN_POINT('',(0.,-0.0107404577624574,-0.00169895351698286));
#24541=CARTESIAN_POINT('Origin',(0.,-0.0090128611052,-0.00596221632729998));
#24542=CARTESIAN_POINT('',(0.,-0.0108005446267269,-0.00126178911315643));
#24543=CARTESIAN_POINT('Origin',(0.,0.,0.));
#24544=CARTESIAN_POINT('Origin',(0.,-0.0102872264807069,0.00330948034739461));
#24545=CARTESIAN_POINT('',(0.,-0.0108717613666412,-0.000220637228970318));
#24546=CARTESIAN_POINT('Origin',(0.,-0.00974076984897448,-0.00467943282721946));
#24547=CARTESIAN_POINT('',(0.,-0.0108717613666412,0.000220637228970165));
#24548=CARTESIAN_POINT('Origin',(0.,0.,0.));
#24549=CARTESIAN_POINT('Origin',(0.,-0.00974076984897455,0.00467943282721932));
#24550=CARTESIAN_POINT('',(0.,-0.0108005446267269,0.00126178911315627));
#24551=CARTESIAN_POINT('Origin',(0.,-0.0102872264807069,-0.00330948034739476));
#24552=CARTESIAN_POINT('',(0.,-0.0107404577624574,0.00169895351698271));
#24553=CARTESIAN_POINT('Origin',(0.,0.,0.));
#24554=CARTESIAN_POINT('Origin',(0.,-0.00901286110520009,0.00596221632729986));
#24555=CARTESIAN_POINT('',(0.,-0.010528134175832,0.00272071071150145));
#24556=CARTESIAN_POINT('Origin',(0.,-0.0106420515472837,-0.00187787851047538));
#24557=CARTESIAN_POINT('',(0.,-0.0104090797518856,0.00314562151551737));
#24558=CARTESIAN_POINT('Origin',(0.,0.,0.));
#24559=CARTESIAN_POINT('Origin',(0.,-0.00811705981202384,0.00713393501814931));
#24560=CARTESIAN_POINT('',(0.,-0.0100596045052361,0.00412895061707371));
#24561=CARTESIAN_POINT('Origin',(0.,-0.0107986353290695,-0.000411295349988447));
#24562=CARTESIAN_POINT('',(0.,-0.00988380028027131,0.00453369253696241));
#24563=CARTESIAN_POINT('Origin',(0.,0.,0.));
#24564=CARTESIAN_POINT('Origin',(0.,-0.00707005305261656,0.00817276199753406));
#24565=CARTESIAN_POINT('',(0.,-0.00940368343621036,0.00546027598492447));
#24566=CARTESIAN_POINT('Origin',(0.,-0.0107540609664773,0.00106294946466809));
#24567=CARTESIAN_POINT('',(0.,-0.0091744043103039,0.00583730944451955));
#24568=CARTESIAN_POINT('Origin',(0.,0.,0.));
#24569=CARTESIAN_POINT('Origin',(0.,-0.00589134458189312,0.00905934588436428));
#24570=CARTESIAN_POINT('',(0.,-0.00857258953722036,0.006689886742415));
#24571=CARTESIAN_POINT('Origin',(0.,-0.0105091587955445,0.00251739354197548));
#24572=CARTESIAN_POINT('',(0.,-0.00829410654667511,0.00703218832173891));
#24573=CARTESIAN_POINT('Origin',(0.,0.,0.));
#24574=CARTESIAN_POINT('Origin',(0.,-0.00460289150846104,0.00977717129830948));
#24575=CARTESIAN_POINT('',(0.,-0.00758180451511425,0.00779487756764615));
#24576=CARTESIAN_POINT('Origin',(0.,-0.0100684908803427,0.00392494334068737));
#24577=CARTESIAN_POINT('',(0.,-0.00725930527113401,0.00809607083593554));
#24578=CARTESIAN_POINT('Origin',(0.,0.,0.));
#24579=CARTESIAN_POINT('Origin',(0.,-0.00322869527523151,0.0103128665100857));
#24580=CARTESIAN_POINT('',(0.,-0.0064497848202166,0.0087546645722668));
#24581=CARTESIAN_POINT('Origin',(0.,-0.00944026603035641,0.00525937887124024));
#24582=CARTESIAN_POINT('',(0.,-0.00608927687352473,0.00900913886881298));
#24583=CARTESIAN_POINT('Origin',(0.,0.,0.));
#24584=CARTESIAN_POINT('Origin',(0.,-0.00179435455795048,0.0106564525314718));
#24585=CARTESIAN_POINT('',(0.,-0.00519761783757985,0.00955136874036762));
#24586=CARTESIAN_POINT('Origin',(0.,-0.0086361868858939,0.00649584212454889));
#24587=CARTESIAN_POINT('',(0.,-0.00480581676911598,0.0097543836905098));
#24588=CARTESIAN_POINT('Origin',(0.,0.,0.));
#24589=CARTESIAN_POINT('Origin',(0.,-0.000326588410304044,0.0108015290049791));
#24590=CARTESIAN_POINT('',(0.,-0.0038486290688996,0.0101701489807191));
#24591=CARTESIAN_POINT('Origin',(0.,-0.00767123192004028,0.00761130012968249));
#24592=CARTESIAN_POINT('',(0.,-0.00343283339125312,0.0103179228000551));
#24593=CARTESIAN_POINT('Origin',(0.,0.,0.));
#24594=CARTESIAN_POINT('Origin',(0.,0.00114726146149736,0.0107453934304013));
#24595=CARTESIAN_POINT('',(0.,-0.0024279476225516,0.0105994785882205));
#24596=CARTESIAN_POINT('Origin',(0.,-0.00656337641804451,0.008584974014533));
#24597=CARTESIAN_POINT('',(0.,-0.00199590282248143,0.0106892585300951));
#24598=CARTESIAN_POINT('Origin',(0.,0.,0.));
#24599=CARTESIAN_POINT('Origin',(0.,0.00259974002297311,0.0104890915072804));
#24600=CARTESIAN_POINT('',(0.,-0.000962038105848782,0.0108313599646072));
#24601=CARTESIAN_POINT('Origin',(0.,-0.00533325763176565,0.00939872607688738));
#24602=CARTESIAN_POINT('Origin',(0.,0.,0.));
#24603=CARTESIAN_POINT('',(0.,0.,-0.009));
#24604=CARTESIAN_POINT('Origin',(0.,0.,0.));
#24605=CARTESIAN_POINT('Origin',(-0.01,0.,0.));
#24606=CARTESIAN_POINT('',(0.006,0.0119602860260496,0.00097547843394005));
#24607=CARTESIAN_POINT('',(0.006,0.0119817149061973,0.000662199295233907));
#24608=CARTESIAN_POINT('Origin',(0.012,0.00974076984897452,-0.00467943282721939));
#24609=CARTESIAN_POINT('',(0.012,0.0108717613666412,-0.000220637228970241));
#24610=CARTESIAN_POINT('Origin',(0.012,0.00974076984897452,0.00467943282721939));
#24611=CARTESIAN_POINT('',(0.012,0.0108717613666412,0.000220637228970242));
#24612=CARTESIAN_POINT('Origin',(0.012,0.,0.));
#24613=CARTESIAN_POINT('Origin',(0.012,0.0102872264807069,-0.00330948034739469));
#24614=CARTESIAN_POINT('',(0.012,0.0108005446267269,0.00126178911315635));
#24615=CARTESIAN_POINT('Origin',(0.012,0.00901286110520005,0.00596221632729992));
#24616=CARTESIAN_POINT('',(0.012,0.0107404577624574,0.00169895351698278));
#24617=CARTESIAN_POINT('Origin',(0.012,0.,0.));
#24618=CARTESIAN_POINT('Origin',(0.012,-0.00400379034671782,-0.0100373976555021));
#24619=CARTESIAN_POINT('',(0.012,0.000521792360520154,-0.0108614735985732));
#24620=CARTESIAN_POINT('Origin',(0.012,0.00533325763176572,-0.00939872607688735));
#24621=CARTESIAN_POINT('',(0.012,0.000962038105848858,-0.0108313599646072));
#24622=CARTESIAN_POINT('Origin',(0.012,0.,0.));
#24623=CARTESIAN_POINT('Origin',(0.012,-0.00259974002297304,-0.0104890915072804));
#24624=CARTESIAN_POINT('',(0.012,0.00199590282248151,-0.0106892585300951));
#24625=CARTESIAN_POINT('Origin',(0.012,0.00656337641804457,-0.00858497401453295));
#24626=CARTESIAN_POINT('',(0.012,0.00242794762255167,-0.0105994785882205));
#24627=CARTESIAN_POINT('Origin',(0.012,0.,0.));
#24628=CARTESIAN_POINT('Origin',(0.012,-0.00114726146149728,-0.0107453934304014));
#24629=CARTESIAN_POINT('',(0.012,0.00343283339125319,-0.0103179228000551));
#24630=CARTESIAN_POINT('Origin',(0.012,0.00767123192004033,-0.00761130012968243));
#24631=CARTESIAN_POINT('',(0.012,0.00384862906889967,-0.010170148980719));
#24632=CARTESIAN_POINT('Origin',(0.012,0.,0.));
#24633=CARTESIAN_POINT('Origin',(0.012,0.00179435455795055,-0.0106564525314718));
#24634=CARTESIAN_POINT('',(0.012,0.00608927687352478,-0.00900913886881295));
#24635=CARTESIAN_POINT('Origin',(0.012,0.00944026603035645,-0.00525937887124018));
#24636=CARTESIAN_POINT('',(0.012,0.00644978482021666,-0.00875466457226676));
#24637=CARTESIAN_POINT('Origin',(0.012,0.,0.));
#24638=CARTESIAN_POINT('Origin',(0.012,0.000326588410304114,-0.0108015290049791));
#24639=CARTESIAN_POINT('',(0.012,0.00480581676911604,-0.00975438369050977));
#24640=CARTESIAN_POINT('Origin',(0.012,0.00863618688589394,-0.00649584212454884));
#24641=CARTESIAN_POINT('',(0.012,0.00519761783757991,-0.00955136874036759));
#24642=CARTESIAN_POINT('Origin',(0.012,0.,0.));
#24643=CARTESIAN_POINT('Origin',(0.012,0.0046028915084611,-0.00977717129830945));
#24644=CARTESIAN_POINT('',(0.012,0.00829410654667516,-0.00703218832173885));
#24645=CARTESIAN_POINT('Origin',(0.012,0.0105091587955445,-0.00251739354197541));
#24646=CARTESIAN_POINT('',(0.012,0.00857258953722041,-0.00668988674241494));
#24647=CARTESIAN_POINT('Origin',(0.012,0.,0.));
#24648=CARTESIAN_POINT('Origin',(0.012,0.00589134458189318,-0.00905934588436424));
#24649=CARTESIAN_POINT('',(0.012,0.00917440431030394,-0.00583730944451949));
#24650=CARTESIAN_POINT('Origin',(0.012,0.0107540609664773,-0.00106294946466802));
#24651=CARTESIAN_POINT('',(0.012,0.0094036834362104,-0.0054602759849244));
#24652=CARTESIAN_POINT('Origin',(0.012,0.,0.));
#24653=CARTESIAN_POINT('Origin',(0.012,0.00322869527523158,-0.0103128665100857));
#24654=CARTESIAN_POINT('',(0.012,0.00725930527113406,-0.00809607083593549));
#24655=CARTESIAN_POINT('Origin',(0.012,0.0100684908803427,-0.0039249433406873));
#24656=CARTESIAN_POINT('',(0.012,0.0075818045151143,-0.0077948775676461));
#24657=CARTESIAN_POINT('Origin',(0.012,0.,0.));
#24658=CARTESIAN_POINT('Origin',(0.012,0.00707005305261661,-0.00817276199753401));
#24659=CARTESIAN_POINT('',(0.012,0.00988380028027134,-0.00453369253696235));
#24660=CARTESIAN_POINT('Origin',(0.012,0.0107986353290695,0.000411295349988523));
#24661=CARTESIAN_POINT('',(0.012,0.0100596045052361,-0.00412895061707364));
#24662=CARTESIAN_POINT('Origin',(0.012,0.,0.));
#24663=CARTESIAN_POINT('Origin',(0.012,0.00811705981202389,-0.00713393501814925));
#24664=CARTESIAN_POINT('',(0.012,0.0104090797518856,-0.0031456215155173));
#24665=CARTESIAN_POINT('Origin',(0.012,0.0106420515472837,0.00187787851047546));
#24666=CARTESIAN_POINT('',(0.012,0.010528134175832,-0.00272071071150138));
#24667=CARTESIAN_POINT('Origin',(0.012,0.,0.));
#24668=CARTESIAN_POINT('Origin',(0.012,0.00901286110520013,-0.00596221632729979));
#24669=CARTESIAN_POINT('',(0.012,0.0107404577624574,-0.00169895351698263));
#24670=CARTESIAN_POINT('Origin',(0.012,0.0102872264807069,0.00330948034739484));
#24671=CARTESIAN_POINT('',(0.012,0.0108005446267269,-0.0012617891131562));
#24672=CARTESIAN_POINT('Origin',(0.012,0.,0.));
#24673=CARTESIAN_POINT('Origin',(0.012,-0.0102872264807069,0.00330948034739461));
#24674=CARTESIAN_POINT('',(0.012,-0.0108005446267269,-0.00126178911315643));
#24675=CARTESIAN_POINT('Origin',(0.012,-0.0090128611052,-0.00596221632729998));
#24676=CARTESIAN_POINT('',(0.012,-0.0107404577624574,-0.00169895351698286));
#24677=CARTESIAN_POINT('Origin',(0.012,0.,0.));
#24678=CARTESIAN_POINT('Origin',(0.012,-0.0106420515472838,0.00187787851047525));
#24679=CARTESIAN_POINT('',(0.012,-0.0105281341758319,-0.00272071071150159));
#24680=CARTESIAN_POINT('Origin',(0.012,-0.00811705981202375,-0.00713393501814942));
#24681=CARTESIAN_POINT('',(0.012,-0.0104090797518855,-0.00314562151551751));
#24682=CARTESIAN_POINT('Origin',(0.012,0.,0.));
#24683=CARTESIAN_POINT('Origin',(0.012,-0.0107986353290695,0.0004112953499883));
#24684=CARTESIAN_POINT('',(0.012,-0.010059604505236,-0.00412895061707385));
#24685=CARTESIAN_POINT('Origin',(0.012,-0.00707005305261645,-0.00817276199753415));
#24686=CARTESIAN_POINT('',(0.012,-0.00988380028027125,-0.00453369253696255));
#24687=CARTESIAN_POINT('Origin',(0.012,0.,0.));
#24688=CARTESIAN_POINT('Origin',(0.012,-0.0105091587955444,-0.00251739354197563));
#24689=CARTESIAN_POINT('',(0.012,-0.00857258953722027,-0.00668988674241512));
#24690=CARTESIAN_POINT('Origin',(0.012,-0.0046028915084609,-0.00977717129830955));
#24691=CARTESIAN_POINT('',(0.012,-0.00829410654667501,-0.00703218832173902));
#24692=CARTESIAN_POINT('Origin',(0.012,0.,0.));
#24693=CARTESIAN_POINT('Origin',(0.012,-0.0107540609664773,-0.00106294946466824));
#24694=CARTESIAN_POINT('',(0.012,-0.00940368343621029,-0.0054602759849246));
#24695=CARTESIAN_POINT('Origin',(0.012,-0.00589134458189299,-0.00905934588436437));
#24696=CARTESIAN_POINT('',(0.012,-0.00917440431030382,-0.00583730944451968));
#24697=CARTESIAN_POINT('Origin',(0.012,0.,0.));
#24698=CARTESIAN_POINT('Origin',(0.012,-0.00944026603035634,-0.00525937887124037));
#24699=CARTESIAN_POINT('',(0.012,-0.00644978482021648,-0.00875466457226689));
#24700=CARTESIAN_POINT('Origin',(0.012,-0.00179435455795034,-0.0106564525314718));
#24701=CARTESIAN_POINT('',(0.012,-0.0060892768735246,-0.00900913886881307));
#24702=CARTESIAN_POINT('Origin',(0.012,0.,0.));
#24703=CARTESIAN_POINT('Origin',(0.012,-0.00863618688589381,-0.00649584212454901));
#24704=CARTESIAN_POINT('',(0.012,-0.00519761783757972,-0.00955136874036769));
#24705=CARTESIAN_POINT('Origin',(0.012,-0.000326588410303897,-0.0108015290049791));
#24706=CARTESIAN_POINT('',(0.012,-0.00480581676911584,-0.00975438369050987));
#24707=CARTESIAN_POINT('Origin',(0.012,0.,0.));
#24708=CARTESIAN_POINT('Origin',(0.012,-0.0100684908803426,-0.00392494334068751));
#24709=CARTESIAN_POINT('',(0.012,-0.00758180451511414,-0.00779487756764626));
#24710=CARTESIAN_POINT('Origin',(0.012,-0.00322869527523136,-0.0103128665100857));
#24711=CARTESIAN_POINT('',(0.012,-0.0072593052711339,-0.00809607083593564));
#24712=CARTESIAN_POINT('Origin',(0.012,0.,0.));
#24713=CARTESIAN_POINT('Origin',(0.012,-0.00767123192004017,-0.00761130012968259));
#24714=CARTESIAN_POINT('',(0.012,-0.00384862906889946,-0.0101701489807191));
#24715=CARTESIAN_POINT('Origin',(0.012,0.0011472614614975,-0.0107453934304013));
#24716=CARTESIAN_POINT('',(0.012,-0.00343283339125298,-0.0103179228000552));
#24717=CARTESIAN_POINT('Origin',(0.012,0.,0.));
#24718=CARTESIAN_POINT('Origin',(0.012,-0.00656337641804439,-0.00858497401453309));
#24719=CARTESIAN_POINT('',(0.012,-0.00242794762255145,-0.0105994785882206));
#24720=CARTESIAN_POINT('Origin',(0.012,0.00259974002297325,-0.0104890915072803));
#24721=CARTESIAN_POINT('',(0.012,-0.00199590282248128,-0.0106892585300951));
#24722=CARTESIAN_POINT('Origin',(0.012,0.,0.));
#24723=CARTESIAN_POINT('Origin',(0.012,-0.00533325763176552,-0.00939872607688746));
#24724=CARTESIAN_POINT('',(0.012,-0.00096203810584863,-0.0108313599646072));
#24725=CARTESIAN_POINT('Origin',(0.012,0.00400379034671803,-0.010037397655502));
#24726=CARTESIAN_POINT('',(0.012,-0.000521792360519925,-0.0108614735985732));
#24727=CARTESIAN_POINT('Origin',(0.012,0.,0.));
#24728=CARTESIAN_POINT('Origin',(0.012,0.00259974002297311,0.0104890915072804));
#24729=CARTESIAN_POINT('',(0.012,-0.00199590282248143,0.0106892585300951));
#24730=CARTESIAN_POINT('Origin',(0.012,-0.00656337641804451,0.008584974014533));
#24731=CARTESIAN_POINT('',(0.012,-0.0024279476225516,0.0105994785882205));
#24732=CARTESIAN_POINT('Origin',(0.012,0.,0.));
#24733=CARTESIAN_POINT('Origin',(0.012,0.00114726146149736,0.0107453934304013));
#24734=CARTESIAN_POINT('',(0.012,-0.00343283339125312,0.0103179228000551));
#24735=CARTESIAN_POINT('Origin',(0.012,-0.00767123192004028,0.00761130012968249));
#24736=CARTESIAN_POINT('',(0.012,-0.0038486290688996,0.0101701489807191));
#24737=CARTESIAN_POINT('Origin',(0.012,0.,0.));
#24738=CARTESIAN_POINT('Origin',(0.012,-0.00179435455795048,0.0106564525314718));
#24739=CARTESIAN_POINT('',(0.012,-0.00608927687352473,0.00900913886881298));
#24740=CARTESIAN_POINT('Origin',(0.012,-0.00944026603035641,0.00525937887124024));
#24741=CARTESIAN_POINT('',(0.012,-0.0064497848202166,0.0087546645722668));
#24742=CARTESIAN_POINT('Origin',(0.012,0.,0.));
#24743=CARTESIAN_POINT('Origin',(0.012,-0.00322869527523151,0.0103128665100857));
#24744=CARTESIAN_POINT('',(0.012,-0.00725930527113401,0.00809607083593554));
#24745=CARTESIAN_POINT('Origin',(0.012,-0.0100684908803427,0.00392494334068737));
#24746=CARTESIAN_POINT('',(0.012,-0.00758180451511425,0.00779487756764615));
#24747=CARTESIAN_POINT('Origin',(0.012,0.,0.));
#24748=CARTESIAN_POINT('Origin',(0.012,-0.000326588410304044,0.0108015290049791));
#24749=CARTESIAN_POINT('',(0.012,-0.00480581676911598,0.0097543836905098));
#24750=CARTESIAN_POINT('Origin',(0.012,-0.0086361868858939,0.00649584212454889));
#24751=CARTESIAN_POINT('',(0.012,-0.00519761783757985,0.00955136874036762));
#24752=CARTESIAN_POINT('Origin',(0.012,0.,0.));
#24753=CARTESIAN_POINT('Origin',(0.012,-0.00707005305261656,0.00817276199753406));
#24754=CARTESIAN_POINT('',(0.012,-0.00988380028027131,0.00453369253696241));
#24755=CARTESIAN_POINT('Origin',(0.012,-0.0107986353290695,-0.000411295349988447));
#24756=CARTESIAN_POINT('',(0.012,-0.0100596045052361,0.00412895061707371));
#24757=CARTESIAN_POINT('Origin',(0.012,0.,0.));
#24758=CARTESIAN_POINT('Origin',(0.012,-0.00589134458189312,0.00905934588436428));
#24759=CARTESIAN_POINT('',(0.012,-0.0091744043103039,0.00583730944451955));
#24760=CARTESIAN_POINT('Origin',(0.012,-0.0107540609664773,0.00106294946466809));
#24761=CARTESIAN_POINT('',(0.012,-0.00940368343621036,0.00546027598492447));
#24762=CARTESIAN_POINT('Origin',(0.012,0.,0.));
#24763=CARTESIAN_POINT('Origin',(0.012,-0.00460289150846104,0.00977717129830948));
#24764=CARTESIAN_POINT('',(0.012,-0.00829410654667511,0.00703218832173891));
#24765=CARTESIAN_POINT('Origin',(0.012,-0.0105091587955445,0.00251739354197548));
#24766=CARTESIAN_POINT('',(0.012,-0.00857258953722036,0.006689886742415));
#24767=CARTESIAN_POINT('Origin',(0.012,0.,0.));
#24768=CARTESIAN_POINT('Origin',(0.012,-0.00811705981202384,0.00713393501814931));
#24769=CARTESIAN_POINT('',(0.012,-0.0104090797518856,0.00314562151551737));
#24770=CARTESIAN_POINT('Origin',(0.012,-0.0106420515472837,-0.00187787851047538));
#24771=CARTESIAN_POINT('',(0.012,-0.010528134175832,0.00272071071150145));
#24772=CARTESIAN_POINT('Origin',(0.012,0.,0.));
#24773=CARTESIAN_POINT('Origin',(0.012,-0.00901286110520009,0.00596221632729986));
#24774=CARTESIAN_POINT('',(0.012,-0.0107404577624574,0.00169895351698271));
#24775=CARTESIAN_POINT('Origin',(0.012,-0.0102872264807069,-0.00330948034739476));
#24776=CARTESIAN_POINT('',(0.012,-0.0108005446267269,0.00126178911315627));
#24777=CARTESIAN_POINT('Origin',(0.012,0.,0.));
#24778=CARTESIAN_POINT('Origin',(0.012,-0.00974076984897455,0.00467943282721932));
#24779=CARTESIAN_POINT('',(0.012,-0.0108717613666412,0.000220637228970165));
#24780=CARTESIAN_POINT('Origin',(0.012,-0.00974076984897448,-0.00467943282721946));
#24781=CARTESIAN_POINT('',(0.012,-0.0108717613666412,-0.000220637228970318));
#24782=CARTESIAN_POINT('Origin',(0.012,0.,0.));
#24783=CARTESIAN_POINT('Origin',(0.012,0.0106420515472837,-0.00187787851047532));
#24784=CARTESIAN_POINT('',(0.012,0.010528134175832,0.00272071071150152));
#24785=CARTESIAN_POINT('Origin',(0.012,0.00811705981202379,0.00713393501814937));
#24786=CARTESIAN_POINT('',(0.012,0.0104090797518855,0.00314562151551744));
#24787=CARTESIAN_POINT('Origin',(0.012,0.,0.));
#24788=CARTESIAN_POINT('Origin',(0.012,0.0107986353290695,-0.000411295349988374));
#24789=CARTESIAN_POINT('',(0.012,0.0100596045052361,0.00412895061707378));
#24790=CARTESIAN_POINT('Origin',(0.012,0.0070700530526165,0.00817276199753411));
#24791=CARTESIAN_POINT('',(0.012,0.00988380028027128,0.00453369253696249));
#24792=CARTESIAN_POINT('Origin',(0.012,0.,0.));
#24793=CARTESIAN_POINT('Origin',(0.012,0.0105091587955444,0.00251739354197556));
#24794=CARTESIAN_POINT('',(0.012,0.00857258953722032,0.00668988674241506));
#24795=CARTESIAN_POINT('Origin',(0.012,0.00460289150846097,0.00977717129830952));
#24796=CARTESIAN_POINT('',(0.012,0.00829410654667506,0.00703218832173896));
#24797=CARTESIAN_POINT('Origin',(0.012,0.,0.));
#24798=CARTESIAN_POINT('Origin',(0.012,0.0100684908803426,0.00392494334068744));
#24799=CARTESIAN_POINT('',(0.012,0.00758180451511419,0.00779487756764621));
#24800=CARTESIAN_POINT('Origin',(0.012,0.00322869527523144,0.0103128665100857));
#24801=CARTESIAN_POINT('',(0.012,0.00725930527113395,0.00809607083593559));
#24802=CARTESIAN_POINT('Origin',(0.012,0.,0.));
#24803=CARTESIAN_POINT('Origin',(0.012,0.0107540609664773,0.00106294946466816));
#24804=CARTESIAN_POINT('',(0.012,0.00940368343621032,0.00546027598492453));
#24805=CARTESIAN_POINT('Origin',(0.012,0.00589134458189306,0.00905934588436432));
#24806=CARTESIAN_POINT('',(0.012,0.00917440431030386,0.00583730944451961));
#24807=CARTESIAN_POINT('Origin',(0.012,0.,0.));
#24808=CARTESIAN_POINT('Origin',(0.012,0.00767123192004022,0.00761130012968254));
#24809=CARTESIAN_POINT('',(0.012,0.00384862906889953,0.0101701489807191));
#24810=CARTESIAN_POINT('Origin',(0.012,-0.00114726146149743,0.0107453934304013));
#24811=CARTESIAN_POINT('',(0.012,0.00343283339125305,0.0103179228000552));
#24812=CARTESIAN_POINT('Origin',(0.012,0.,0.));
#24813=CARTESIAN_POINT('Origin',(0.012,0.00863618688589385,0.00649584212454895));
#24814=CARTESIAN_POINT('',(0.012,0.00519761783757978,0.00955136874036766));
#24815=CARTESIAN_POINT('Origin',(0.012,0.00032658841030397,0.0108015290049791));
#24816=CARTESIAN_POINT('',(0.012,0.00480581676911591,0.00975438369050984));
#24817=CARTESIAN_POINT('Origin',(0.012,0.,0.));
#24818=CARTESIAN_POINT('Origin',(0.012,0.00944026603035638,0.00525937887124031));
#24819=CARTESIAN_POINT('',(0.012,0.00644978482021654,0.00875466457226685));
#24820=CARTESIAN_POINT('Origin',(0.012,0.00179435455795041,0.0106564525314718));
#24821=CARTESIAN_POINT('',(0.012,0.00608927687352466,0.00900913886881303));
#24822=CARTESIAN_POINT('Origin',(0.012,0.,0.));
#24823=CARTESIAN_POINT('Origin',(0.012,0.00656337641804445,0.00858497401453304));
#24824=CARTESIAN_POINT('',(0.012,0.00242794762255152,0.0105994785882206));
#24825=CARTESIAN_POINT('Origin',(0.012,-0.00259974002297318,0.0104890915072804));
#24826=CARTESIAN_POINT('',(0.012,0.00199590282248136,0.0106892585300951));
#24827=CARTESIAN_POINT('Origin',(0.012,0.,0.));
#24828=CARTESIAN_POINT('Origin',(0.012,0.00533325763176559,0.00939872607688742));
#24829=CARTESIAN_POINT('',(0.012,0.000962038105848705,0.0108313599646072));
#24830=CARTESIAN_POINT('Origin',(0.012,-0.00400379034671796,0.010037397655502));
#24831=CARTESIAN_POINT('',(0.012,0.000521792360520001,0.0108614735985732));
#24832=CARTESIAN_POINT('Origin',(0.012,0.,0.));
#24833=CARTESIAN_POINT('Origin',(0.012,0.00400379034671789,0.010037397655502));
#24834=CARTESIAN_POINT('',(0.012,-0.000521792360520078,0.0108614735985732));
#24835=CARTESIAN_POINT('Origin',(0.012,-0.00533325763176565,0.00939872607688738));
#24836=CARTESIAN_POINT('',(0.012,-0.000962038105848782,0.0108313599646072));
#24837=CARTESIAN_POINT('Origin',(0.012,0.,0.));
#24838=CARTESIAN_POINT('Origin',(0.0500000508,0.,0.));
#24839=CARTESIAN_POINT('',(0.0500000508,-1.10218211923262E-18,-0.009));
#54550=UNCERTAINTY_MEASURE_WITH_UNIT(LENGTH_MEASURE(1.E-5),#54581,
'DISTANCE_ACCURACY_VALUE',
'Maximum model space distance between geometric entities at asserted c
onnectivities');
#54564=UNCERTAINTY_MEASURE_WITH_UNIT(LENGTH_MEASURE(1.E-5),#54581,
'DISTANCE_ACCURACY_VALUE',
'Maximum model space distance between geometric entities at asserted c
onnectivities');
#54566=(
GEOMETRIC_REPRESENTATION_CONTEXT(3)
GLOBAL_UNCERTAINTY_ASSIGNED_CONTEXT((#54550))
GLOBAL_UNIT_ASSIGNED_CONTEXT((#54581,#54582,#54583))
REPRESENTATION_CONTEXT('','3D')
);
#54580=(
GEOMETRIC_REPRESENTATION_CONTEXT(3)
GLOBAL_UNCERTAINTY_ASSIGNED_CONTEXT((#54564))
GLOBAL_UNIT_ASSIGNED_CONTEXT((#54581,#54582,#54583))
REPRESENTATION_CONTEXT('','3D')
);
#54581=(
LENGTH_UNIT()
NAMED_UNIT(*)
SI_UNIT($,.METRE.)
);
#54582=(
NAMED_UNIT(*)
PLANE_ANGLE_UNIT()
SI_UNIT($,.RADIAN.)
);
#54583=(
NAMED_UNIT(*)
SI_UNIT($,.STERADIAN.)
SOLID_ANGLE_UNIT()
);
#54585=SHAPE_DEFINITION_REPRESENTATION(#54600,#54630);
#54600=PRODUCT_DEFINITION_SHAPE('',$,#54646);
#54630=SHAPE_REPRESENTATION('',(#17836),#54566);
#54644=PRODUCT_DEFINITION_CONTEXT('part definition',#54691,'design');
#54646=PRODUCT_DEFINITION('Part_7','Part_7',#54661,#54644);
#54661=PRODUCT_DEFINITION_FORMATION('',$,#54694);
#54691=APPLICATION_CONTEXT(
'Core Data for Automotive Mechanical Design Process');
#54692=PRODUCT_CONTEXT('part definition',#54691,'mechanical');
#54694=PRODUCT('Part_7','Part_7','Part 1',(#54692));
#54709=PRESENTATION_STYLE_ASSIGNMENT((#54719));
#54719=SURFACE_STYLE_USAGE(.BOTH.,#54729);
#54729=SURFACE_SIDE_STYLE('',(#54739));
#54739=SURFACE_STYLE_FILL_AREA(#54749);
#54749=FILL_AREA_STYLE('Opaque(153,153,153)',(#54759));
#54759=FILL_AREA_STYLE_COLOUR('Opaque(153,153,153)',#54769);
#54769=COLOUR_RGB('Opaque(153,153,153)', 0.09019608, 0.27058824, 0.51372549);
ENDSEC;
END-ISO-10303-21;
